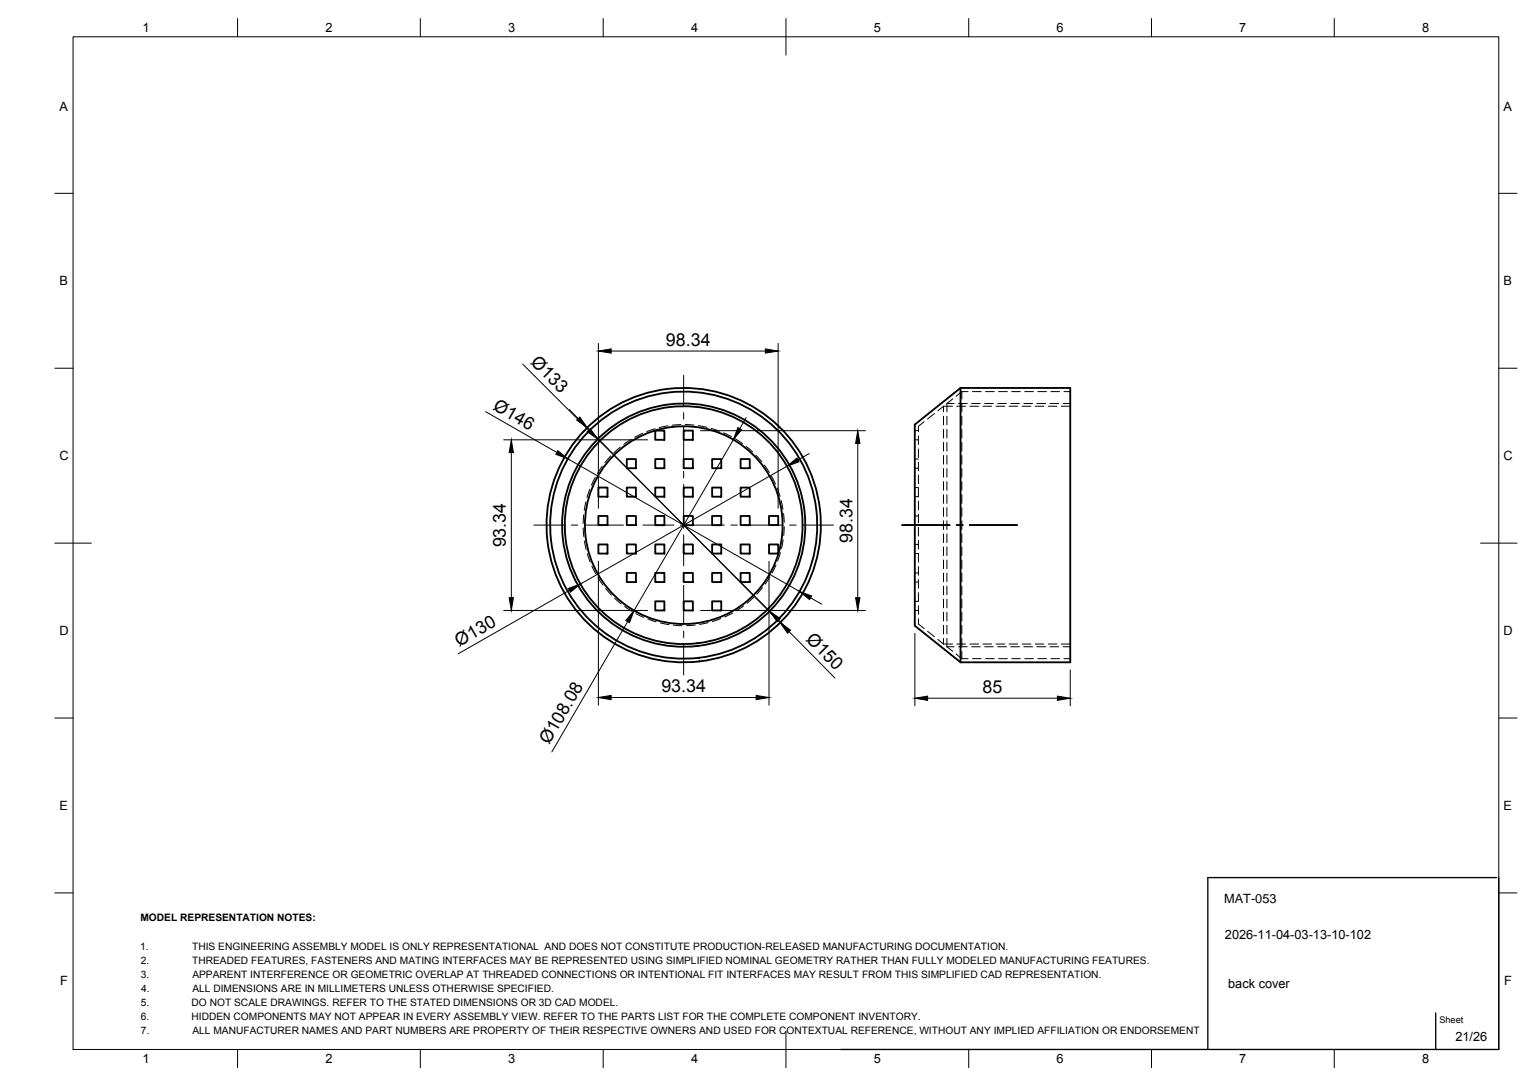
ISO-10303-21;
HEADER;
FILE_DESCRIPTION (('STEP AP214'),
    '1' );
FILE_NAME ('back cover.step',
    '2026-10-10T03:43:58',
    ( '' ),
    ( '' ),
    'SwSTEP 2.0',
    'SolidWorks 2026',
    '' );
FILE_SCHEMA (( 'AUTOMOTIVE_DESIGN' ));
ENDSEC;

DATA;
#6=DIRECTION ( 'NONE',  ( 0.000000000000000000, -1.000000000000000000, 0.000000000000000000 ) ) ;
#36=CARTESIAN_POINT ( 'NONE',  ( 0.000000000000000000, 0.000000000000000000, 0.000000000000000000 ) ) ;
#57=AXIS2_PLACEMENT_3D ( 'NONE', #19183, #8994, #35375 ) ;
#63=ORIENTED_EDGE ( 'NONE', *, *, #15028, .F. ) ;
#64=ORIENTED_EDGE ( 'NONE', *, *, #47335, .F. ) ;
#74=VECTOR ( 'NONE', #64267, 1000.000000000000000 ) ;
#81=CARTESIAN_POINT ( 'NONE',  ( -20.55634918610396866, 36.11269837220808654, 0.000000000000000000 ) ) ;
#91=CARTESIAN_POINT ( 'NONE',  ( 0.000000000000000000, 0.000000000000000000, 25.00000000000007816 ) ) ;
#96=DIRECTION ( 'NONE',  ( -0.000000000000000000, -0.000000000000000000, -1.000000000000000000 ) ) ;
#97=ORIENTED_EDGE ( 'NONE', *, *, #54272, .F. ) ;
#104=VECTOR ( 'NONE', #8568, 1000.000000000000000 ) ;
#111=VECTOR ( 'NONE', #38454, 1000.000000000000000 ) ;
#118=DIRECTION ( 'NONE',  ( -0.000000000000000000, -0.000000000000000000, -1.000000000000000000 ) ) ;
#120=ORIENTED_EDGE ( 'NONE', *, *, #64988, .T. ) ;
#150=EDGE_CURVE ( 'NONE', #43731, #18069, #10487, .T. ) ;
#166=AXIS2_PLACEMENT_3D ( 'NONE', #40198, #13463, #28960 ) ;
#171=VECTOR ( 'NONE', #36242, 1000.000000000000000 ) ;
#190=CARTESIAN_POINT ( 'NONE',  ( -31.11269837220812207, -26.11269837220801193, 0.000000000000000000 ) ) ;
#192=VERTEX_POINT ( 'NONE', #42509 ) ;
#195=FACE_BOUND ( 'NONE', #48020, .T. ) ;
#204=LINE ( 'NONE', #41148, #41347 ) ;
#234=EDGE_CURVE ( 'NONE', #1187, #8293, #15089, .T. ) ;
#287=LINE ( 'NONE', #43194, #50190 ) ;
#293=ORIENTED_EDGE ( 'NONE', *, *, #14607, .T. ) ;
#296=VECTOR ( 'NONE', #1863, 1000.000000000000000 ) ;
#300=FACE_OUTER_BOUND ( 'NONE', #57072, .T. ) ;
#306=AXIS2_PLACEMENT_3D ( 'NONE', #41965, #53186, #58819 ) ;
#322=ADVANCED_FACE ( 'NONE', ( #635 ), #43872, .F. ) ;
#327=VERTEX_POINT ( 'NONE', #60057 ) ;
#344=VECTOR ( 'NONE', #34891, 1000.000000000000000 ) ;
#349=DIRECTION ( 'NONE',  ( -1.000000000000000000, 0.000000000000000000, 0.000000000000000000 ) ) ;
#371=CARTESIAN_POINT ( 'NONE',  ( -20.55634918610396866, 31.11269837220809009, 0.000000000000000000 ) ) ;
#418=AXIS2_PLACEMENT_3D ( 'NONE', #49039, #43423, #65240 ) ;
#430=CARTESIAN_POINT ( 'NONE',  ( -20.55634918610403261, 0.000000000000000000, 2.000000000000000000 ) ) ;
#437=DIRECTION ( 'NONE',  ( 0.000000000000000000, 0.000000000000000000, 1.000000000000000000 ) ) ;
#440=DIRECTION ( 'NONE',  ( 0.000000000000000000, 1.000000000000000000, 0.000000000000000000 ) ) ;
#447=ORIENTED_EDGE ( 'NONE', *, *, #56885, .F. ) ;
#455=CARTESIAN_POINT ( 'NONE',  ( 15.55634918610400241, -15.55634918610406103, 85.00100000000000477 ) ) ;
#465=AXIS2_PLACEMENT_3D ( 'NONE', #65616, #23741, #6150 ) ;
#481=DIRECTION ( 'NONE',  ( 0.000000000000000000, 0.000000000000000000, 1.000000000000000000 ) ) ;
#522=VECTOR ( 'NONE', #50610, 1000.000000000000000 ) ;
#544=CARTESIAN_POINT ( 'NONE',  ( 6.375108774214766072E-14, 31.11269837220806167, 0.000000000000000000 ) ) ;
#553=CARTESIAN_POINT ( 'NONE',  ( -2.645453300864630819E-14, -15.55634918610403616, 2.000000000000001776 ) ) ;
#556=ADVANCED_FACE ( 'NONE', ( #43363 ), #46664, .F. ) ;
#557=DIRECTION ( 'NONE',  ( 0.000000000000000000, 1.000000000000000000, -0.000000000000000000 ) ) ;
#558=VECTOR ( 'NONE', #9205, 1000.000000000000000 ) ;
#565=LINE ( 'NONE', #27282, #37965 ) ;
#576=EDGE_LOOP ( 'NONE', ( #32786, #49878, #58567, #41798 ) ) ;
#578=CARTESIAN_POINT ( 'NONE',  ( -15.55634918610405748, -15.55634918610400774, 85.00100000000000477 ) ) ;
#588=EDGE_LOOP ( 'NONE', ( #66796, #38550, #24211, #31113 ) ) ;
#600=CARTESIAN_POINT ( 'NONE',  ( -7.329206686002009974E-14, -46.66904755831211560, 85.00100000000000477 ) ) ;
#607=ORIENTED_EDGE ( 'NONE', *, *, #30585, .F. ) ;
#613=EDGE_CURVE ( 'NONE', #67838, #27835, #64835, .T. ) ;
#632=EDGE_CURVE ( 'NONE', #26921, #4856, #48977, .T. ) ;
#635=FACE_OUTER_BOUND ( 'NONE', #24714, .T. ) ;
#643=ORIENTED_EDGE ( 'NONE', *, *, #36304, .T. ) ;
#661=DIRECTION ( 'NONE',  ( 0.000000000000000000, -1.000000000000000000, 0.000000000000000000 ) ) ;
#666=LINE ( 'NONE', #15804, #31702 ) ;
#730=FACE_OUTER_BOUND ( 'NONE', #7347, .T. ) ;
#790=EDGE_CURVE ( 'NONE', #8416, #11547, #57246, .T. ) ;
#801=ORIENTED_EDGE ( 'NONE', *, *, #53338, .F. ) ;
#827=DIRECTION ( 'NONE',  ( 0.000000000000000000, -1.000000000000000000, 0.000000000000000000 ) ) ;
#828=FACE_OUTER_BOUND ( 'NONE', #18462, .T. ) ;
#840=ORIENTED_EDGE ( 'NONE', *, *, #43108, .F. ) ;
#841=CARTESIAN_POINT ( 'NONE',  ( 0.000000000000000000, 0.000000000000000000, 85.00000000000000000 ) ) ;
#848=VECTOR ( 'NONE', #5552, 1000.000000000000000 ) ;
#877=ORIENTED_EDGE ( 'NONE', *, *, #51299, .F. ) ;
#882=DIRECTION ( 'NONE',  ( 0.000000000000000000, 1.000000000000000000, 0.000000000000000000 ) ) ;
#885=ORIENTED_EDGE ( 'NONE', *, *, #41118, .F. ) ;
#888=ORIENTED_EDGE ( 'NONE', *, *, #62836, .F. ) ;
#891=FACE_OUTER_BOUND ( 'NONE', #1268, .T. ) ;
#904=PLANE ( 'NONE',  #39037 ) ;
#906=DIRECTION ( 'NONE',  ( 1.000000000000000000, -0.000000000000000000, -0.000000000000000000 ) ) ;
#913=VERTEX_POINT ( 'NONE', #44161 ) ;
#920=CARTESIAN_POINT ( 'NONE',  ( 15.55634918610411610, 46.66904755831205875, 85.00100000000000477 ) ) ;
#931=DIRECTION ( 'NONE',  ( -1.000000000000000000, 0.000000000000000000, 0.000000000000000000 ) ) ;
#949=DIRECTION ( 'NONE',  ( 0.000000000000000000, 1.000000000000000000, -0.000000000000000000 ) ) ;
#958=VECTOR ( 'NONE', #53885, 1000.000000000000000 ) ;
#975=DIRECTION ( 'NONE',  ( 0.000000000000000000, 1.000000000000000000, -0.000000000000000000 ) ) ;
#984=CARTESIAN_POINT ( 'NONE',  ( -5.000000000000073719, -41.66904755831212270, 0.000000000000000000 ) ) ;
#993=ORIENTED_EDGE ( 'NONE', *, *, #35206, .T. ) ;
#1007=VECTOR ( 'NONE', #24608, 1000.000000000000000 ) ;
#1009=EDGE_CURVE ( 'NONE', #57581, #8542, #59993, .T. ) ;
#1021=EDGE_LOOP ( 'NONE', ( #20694, #3514, #16394, #42951 ) ) ;
#1035=VERTEX_POINT ( 'NONE', #14260 ) ;
#1047=CARTESIAN_POINT ( 'NONE',  ( 31.11269837220803325, -15.55634918610409656, 2.000000000000001776 ) ) ;
#1053=LINE ( 'NONE', #32712, #68406 ) ;
#1066=ORIENTED_EDGE ( 'NONE', *, *, #15157, .T. ) ;
#1079=CARTESIAN_POINT ( 'NONE',  ( -4.999999999999936939, 36.11269837220805812, 85.00100000000000477 ) ) ;
#1083=LINE ( 'NONE', #49599, #33421 ) ;
#1087=CARTESIAN_POINT ( 'NONE',  ( -51.66904755831212981, -15.55634918610397222, 0.000000000000000000 ) ) ;
#1089=ORIENTED_EDGE ( 'NONE', *, *, #65531, .F. ) ;
#1090=VECTOR ( 'NONE', #39346, 1000.000000000000000 ) ;
#1106=ORIENTED_EDGE ( 'NONE', *, *, #20088, .F. ) ;
#1122=LINE ( 'NONE', #17650, #64641 ) ;
#1141=LINE ( 'NONE', #39137, #57724 ) ;
#1164=EDGE_CURVE ( 'NONE', #53174, #39681, #69076, .T. ) ;
#1173=VECTOR ( 'NONE', #25176, 1000.000000000000000 ) ;
#1177=CARTESIAN_POINT ( 'NONE',  ( 10.55634918610400419, -10.55634918610406281, 2.000000000000001776 ) ) ;
#1178=LINE ( 'NONE', #22633, #24273 ) ;
#1187=VERTEX_POINT ( 'NONE', #69435 ) ;
#1190=SURFACE_STYLE_FILL_AREA ( #60284 ) ;
#1192=EDGE_CURVE ( 'NONE', #19369, #63634, #42702, .T. ) ;
#1203=DIRECTION ( 'NONE',  ( -1.000000000000000000, 0.000000000000000000, 0.000000000000000000 ) ) ;
#1226=CARTESIAN_POINT ( 'NONE',  ( -31.11269837220801193, 31.11269837220812207, 2.000000000000001776 ) ) ;
#1235=VERTEX_POINT ( 'NONE', #11731 ) ;
#1248=FACE_OUTER_BOUND ( 'NONE', #33448, .T. ) ;
#1249=ADVANCED_FACE ( 'NONE', ( #66278 ), #33203, .F. ) ;
#1250=FACE_BOUND ( 'NONE', #49319, .T. ) ;
#1268=EDGE_LOOP ( 'NONE', ( #11768, #41933, #16549, #1900 ) ) ;
#1271=VECTOR ( 'NONE', #7727, 1000.000000000000000 ) ;
#1283=EDGE_LOOP ( 'NONE', ( #47982, #4355, #44982, #36285 ) ) ;
#1293=DIRECTION ( 'NONE',  ( 1.000000000000000000, -0.000000000000000000, 0.000000000000000000 ) ) ;
#1326=PLANE ( 'NONE',  #5078 ) ;
#1335=VECTOR ( 'NONE', #46755, 1000.000000000000000 ) ;
#1344=DIRECTION ( 'NONE',  ( -0.000000000000000000, -0.000000000000000000, -1.000000000000000000 ) ) ;
#1346=DIRECTION ( 'NONE',  ( 1.000000000000000000, -0.000000000000000000, 0.000000000000000000 ) ) ;
#1349=EDGE_CURVE ( 'NONE', #50750, #8416, #55694, .T. ) ;
#1351=ORIENTED_EDGE ( 'NONE', *, *, #50161, .T. ) ;
#1361=DIRECTION ( 'NONE',  ( 0.000000000000000000, 0.000000000000000000, 1.000000000000000000 ) ) ;
#1381=EDGE_LOOP ( 'NONE', ( #20943, #1491, #51722, #43619 ) ) ;
#1386=AXIS2_PLACEMENT_3D ( 'NONE', #23783, #34697, #56132 ) ;
#1398=PLANE ( 'NONE',  #59758 ) ;
#1420=CARTESIAN_POINT ( 'NONE',  ( 10.55634918610400419, -15.55634918610406103, 85.00100000000000477 ) ) ;
#1446=DIRECTION ( 'NONE',  ( 1.000000000000000000, 0.000000000000000000, 0.000000000000000000 ) ) ;
#1451=CARTESIAN_POINT ( 'NONE',  ( -20.55634918610405748, -15.55634918610400774, 0.000000000000000000 ) ) ;
#1454=VERTEX_POINT ( 'NONE', #29656 ) ;
#1459=DIRECTION ( 'NONE',  ( 0.000000000000000000, -1.000000000000000000, 0.000000000000000000 ) ) ;
#1467=CARTESIAN_POINT ( 'NONE',  ( 41.66904755831212981, 15.55634918610394379, 0.000000000000000000 ) ) ;
#1482=ORIENTED_EDGE ( 'NONE', *, *, #22147, .F. ) ;
#1491=ORIENTED_EDGE ( 'NONE', *, *, #22147, .T. ) ;
#1534=ORIENTED_EDGE ( 'NONE', *, *, #38769, .T. ) ;
#1544=ORIENTED_EDGE ( 'NONE', *, *, #54272, .T. ) ;
#1582=DIRECTION ( 'NONE',  ( -0.000000000000000000, -1.000000000000000000, -0.000000000000000000 ) ) ;
#1608=CARTESIAN_POINT ( 'NONE',  ( 15.55634918610397399, -26.11269837220809364, 2.000000000000001776 ) ) ;
#1617=VERTEX_POINT ( 'NONE', #5168 ) ;
#1620=CARTESIAN_POINT ( 'NONE',  ( 10.55634918610411432, 51.66904755831205875, 85.00100000000000477 ) ) ;
#1635=LINE ( 'NONE', #12540, #16170 ) ;
#1653=ORIENTED_EDGE ( 'NONE', *, *, #26539, .T. ) ;
#1656=CARTESIAN_POINT ( 'NONE',  ( 31.11269837220800127, -31.11269837220812562, 2.000000000000001776 ) ) ;
#1657=DIRECTION ( 'NONE',  ( 0.000000000000000000, -0.000000000000000000, -1.000000000000000000 ) ) ;
#1672=AXIS2_PLACEMENT_3D ( 'NONE', #56432, #23047, #8255 ) ;
#1674=EDGE_CURVE ( 'NONE', #9968, #27957, #11131, .T. ) ;
#1729=DIRECTION ( 'NONE',  ( -0.000000000000000000, -0.000000000000000000, -1.000000000000000000 ) ) ;
#1731=ORIENTED_EDGE ( 'NONE', *, *, #59531, .F. ) ;
#1738=ORIENTED_EDGE ( 'NONE', *, *, #8963, .F. ) ;
#1759=ADVANCED_FACE ( 'NONE', ( #12190 ), #60716, .F. ) ;
#1764=DIRECTION ( 'NONE',  ( 0.000000000000000000, 0.000000000000000000, 1.000000000000000000 ) ) ;
#1768=EDGE_CURVE ( 'NONE', #27095, #38528, #55793, .T. ) ;
#1790=LINE ( 'NONE', #17961, #25329 ) ;
#1818=CARTESIAN_POINT ( 'NONE',  ( -5.767955557622883589E-14, -26.11269837220806522, 2.000000000000001776 ) ) ;
#1826=EDGE_CURVE ( 'NONE', #31701, #24549, #49803, .T. ) ;
#1853=DIRECTION ( 'NONE',  ( -1.000000000000000000, 0.000000000000000000, 0.000000000000000000 ) ) ;
#1863=DIRECTION ( 'NONE',  ( 0.000000000000000000, -1.000000000000000000, 0.000000000000000000 ) ) ;
#1888=VECTOR ( 'NONE', #8941, 1000.000000000000000 ) ;
#1894=CARTESIAN_POINT ( 'NONE',  ( 41.66904755831210849, -9.150666335777657423E-14, 85.00100000000000477 ) ) ;
#1900=ORIENTED_EDGE ( 'NONE', *, *, #46935, .F. ) ;
#1904=ORIENTED_EDGE ( 'NONE', *, *, #36060, .T. ) ;
#1909=EDGE_CURVE ( 'NONE', #62027, #63672, #20228, .T. ) ;
#1915=EDGE_CURVE ( 'NONE', #26889, #39680, #35031, .T. ) ;
#1916=ORIENTED_EDGE ( 'NONE', *, *, #8825, .T. ) ;
#1997=ORIENTED_EDGE ( 'NONE', *, *, #12232, .T. ) ;
#2018=VERTEX_POINT ( 'NONE', #25866 ) ;
#2020=CARTESIAN_POINT ( 'NONE',  ( 10.55634918610411432, 46.66904755831205875, 85.00100000000000477 ) ) ;
#2021=DIRECTION ( 'NONE',  ( -1.000000000000000000, 0.000000000000000000, 0.000000000000000000 ) ) ;
#2046=DIRECTION ( 'NONE',  ( -1.000000000000000000, 0.000000000000000000, 0.000000000000000000 ) ) ;
#2084=EDGE_CURVE ( 'NONE', #40853, #60572, #12105, .T. ) ;
#2088=ORIENTED_EDGE ( 'NONE', *, *, #49767, .F. ) ;
#2106=DIRECTION ( 'NONE',  ( 0.000000000000000000, -1.000000000000000000, 0.000000000000000000 ) ) ;
#2109=DIRECTION ( 'NONE',  ( 1.000000000000000000, -0.000000000000000000, 0.000000000000000000 ) ) ;
#2113=DIRECTION ( 'NONE',  ( -0.000000000000000000, -0.000000000000000000, -1.000000000000000000 ) ) ;
#2161=ORIENTED_EDGE ( 'NONE', *, *, #63382, .T. ) ;
#2162=LINE ( 'NONE', #13743, #57665 ) ;
#2168=LINE ( 'NONE', #45410, #29903 ) ;
#2172=EDGE_LOOP ( 'NONE', ( #17537, #12775, #56513, #41341 ) ) ;
#2175=LINE ( 'NONE', #18695, #68256 ) ;
#2187=DIRECTION ( 'NONE',  ( -1.000000000000000000, 0.000000000000000000, 0.000000000000000000 ) ) ;
#2188=DIRECTION ( 'NONE',  ( -1.000000000000000000, 0.000000000000000000, 0.000000000000000000 ) ) ;
#2213=LINE ( 'NONE', #32821, #63921 ) ;
#2216=ORIENTED_EDGE ( 'NONE', *, *, #20941, .T. ) ;
#2224=VECTOR ( 'NONE', #64142, 1000.000000000000000 ) ;
#2257=ORIENTED_EDGE ( 'NONE', *, *, #26764, .T. ) ;
#2258=PLANE ( 'NONE',  #31609 ) ;
#2265=CARTESIAN_POINT ( 'NONE',  ( -46.66904755831212981, -15.55634918610397222, 0.000000000000000000 ) ) ;
#2333=PLANE ( 'NONE',  #1386 ) ;
#2344=LINE ( 'NONE', #17101, #4229 ) ;
#2345=VECTOR ( 'NONE', #16431, 1000.000000000000000 ) ;
#2361=VECTOR ( 'NONE', #29823, 1000.000000000000000 ) ;
#2391=FACE_BOUND ( 'NONE', #20555, .T. ) ;
#2401=EDGE_CURVE ( 'NONE', #58133, #49065, #24667, .T. ) ;
#2426=CARTESIAN_POINT ( 'NONE',  ( 15.55634918610400241, -15.55634918610406103, 0.000000000000000000 ) ) ;
#2442=VECTOR ( 'NONE', #25225, 1000.000000000000000 ) ;
#2449=DIRECTION ( 'NONE',  ( 1.000000000000000000, -0.000000000000000000, 0.000000000000000000 ) ) ;
#2473=ORIENTED_EDGE ( 'NONE', *, *, #43442, .T. ) ;
#2482=EDGE_LOOP ( 'NONE', ( #8029, #97, #20347, #42967 ) ) ;
#2498=VECTOR ( 'NONE', #34813, 1000.000000000000000 ) ;
#2500=ORIENTED_EDGE ( 'NONE', *, *, #27204, .T. ) ;
#2502=ORIENTED_EDGE ( 'NONE', *, *, #48803, .F. ) ;
#2504=CIRCLE ( 'NONE', #11457, 66.50000000000000000 ) ;
#2517=CARTESIAN_POINT ( 'NONE',  ( -5.000000000000073719, -41.66904755831212270, 85.00100000000000477 ) ) ;
#2519=FACE_OUTER_BOUND ( 'NONE', #35690, .T. ) ;
#2538=ORIENTED_EDGE ( 'NONE', *, *, #32611, .T. ) ;
#2539=CARTESIAN_POINT ( 'NONE',  ( -5.767955557622883589E-14, -31.11269837220806878, 0.000000000000000000 ) ) ;
#2540=ADVANCED_FACE ( 'NONE', ( #63328 ), #42214, .F. ) ;
#2545=LINE ( 'NONE', #8521, #51988 ) ;
#2550=ORIENTED_EDGE ( 'NONE', *, *, #27368, .F. ) ;
#2570=ORIENTED_EDGE ( 'NONE', *, *, #11979, .T. ) ;
#2579=FACE_OUTER_BOUND ( 'NONE', #67824, .T. ) ;
#2590=CARTESIAN_POINT ( 'NONE',  ( 41.66904755831210849, 4.999999999999909406, 2.000000000000001776 ) ) ;
#2629=PLANE ( 'NONE',  #1672 ) ;
#2631=DIRECTION ( 'NONE',  ( -1.000000000000000000, 0.000000000000000000, 0.000000000000000000 ) ) ;
#2645=PLANE ( 'NONE',  #51441 ) ;
#2651=VERTEX_POINT ( 'NONE', #22484 ) ;
#2660=DIRECTION ( 'NONE',  ( -0.000000000000000000, -0.000000000000000000, -1.000000000000000000 ) ) ;
#2670=LINE ( 'NONE', #30103, #1173 ) ;
#2689=ORIENTED_EDGE ( 'NONE', *, *, #47335, .T. ) ;
#2701=VECTOR ( 'NONE', #8433, 1000.000000000000000 ) ;
#2704=VECTOR ( 'NONE', #14100, 999.9999999999998863 ) ;
#2716=ORIENTED_EDGE ( 'NONE', *, *, #45081, .F. ) ;
#2723=LINE ( 'NONE', #35425, #51095 ) ;
#2726=ORIENTED_EDGE ( 'NONE', *, *, #15157, .F. ) ;
#2732=ORIENTED_EDGE ( 'NONE', *, *, #31234, .T. ) ;
#2735=FACE_BOUND ( 'NONE', #45270, .T. ) ;
#2736=VECTOR ( 'NONE', #37672, 1000.000000000000000 ) ;
#2764=FACE_OUTER_BOUND ( 'NONE', #14655, .T. ) ;
#2783=VECTOR ( 'NONE', #29904, 1000.000000000000000 ) ;
#2789=CARTESIAN_POINT ( 'NONE',  ( -31.11269837220801193, 31.11269837220812207, 2.000000000000001776 ) ) ;
#2803=CARTESIAN_POINT ( 'NONE',  ( 15.55634918610411610, 46.66904755831205875, 0.000000000000000000 ) ) ;
#2836=DIRECTION ( 'NONE',  ( -1.000000000000000000, 0.000000000000000000, 0.000000000000000000 ) ) ;
#2837=EDGE_CURVE ( 'NONE', #34252, #12488, #63161, .T. ) ;
#2847=AXIS2_PLACEMENT_3D ( 'NONE', #55235, #19692, #19004 ) ;
#2860=ADVANCED_FACE ( 'NONE', ( #52591 ), #57538, .F. ) ;
#2864=CARTESIAN_POINT ( 'NONE',  ( -20.55634918610403261, 5.000000000000028422, 85.00100000000000477 ) ) ;
#2865=ADVANCED_FACE ( 'NONE', ( #24240 ), #28817, .F. ) ;
#2871=CARTESIAN_POINT ( 'NONE',  ( 31.11269837220806522, -6.375108774214766072E-14, 0.000000000000000000 ) ) ;
#2886=AXIS2_PLACEMENT_3D ( 'NONE', #12370, #66210, #45064 ) ;
#2899=DIRECTION ( 'NONE',  ( -0.000000000000000000, -0.000000000000000000, -1.000000000000000000 ) ) ;
#2908=PLANE ( 'NONE',  #63965 ) ;
#2921=CARTESIAN_POINT ( 'NONE',  ( -5.767955557622883589E-14, -26.11269837220806522, 0.000000000000000000 ) ) ;
#2924=DIRECTION ( 'NONE',  ( 1.000000000000000000, 0.000000000000000000, 0.000000000000000000 ) ) ;
#2926=EDGE_CURVE ( 'NONE', #61056, #43813, #64883, .T. ) ;
#2998=CARTESIAN_POINT ( 'NONE',  ( 46.66904755831207297, -15.55634918610412853, 85.00100000000000477 ) ) ;
#3003=DIRECTION ( 'NONE',  ( 0.000000000000000000, -1.000000000000000000, 0.000000000000000000 ) ) ;
#3006=ORIENTED_EDGE ( 'NONE', *, *, #12801, .T. ) ;
#3014=EDGE_CURVE ( 'NONE', #26941, #30210, #39202, .T. ) ;
#3043=DIRECTION ( 'NONE',  ( -0.000000000000000000, -0.000000000000000000, -1.000000000000000000 ) ) ;
#3073=LINE ( 'NONE', #24536, #42722 ) ;
#3074=LINE ( 'NONE', #56888, #2442 ) ;
#3090=ORIENTED_EDGE ( 'NONE', *, *, #38328, .F. ) ;
#3093=ADVANCED_FACE ( 'NONE', ( #8228 ), #9260, .F. ) ;
#3094=AXIS2_PLACEMENT_3D ( 'NONE', #16311, #33194, #481 ) ;
#3103=DIRECTION ( 'NONE',  ( 0.000000000000000000, 1.000000000000000000, 0.000000000000000000 ) ) ;
#3141=AXIS2_PLACEMENT_3D ( 'NONE', #68861, #20685, #1657 ) ;
#3154=DIRECTION ( 'NONE',  ( -0.000000000000000000, -0.000000000000000000, -1.000000000000000000 ) ) ;
#3173=EDGE_CURVE ( 'NONE', #53918, #30808, #10975, .T. ) ;
#3178=ADVANCED_FACE ( 'NONE', ( #37029 ), #47913, .F. ) ;
#3196=DIRECTION ( 'NONE',  ( 0.000000000000000000, 0.000000000000000000, 1.000000000000000000 ) ) ;
#3198=ORIENTED_EDGE ( 'NONE', *, *, #22337, .F. ) ;
#3216=CARTESIAN_POINT ( 'NONE',  ( -15.55634918610400597, 15.55634918610405748, 85.00100000000000477 ) ) ;
#3219=DIRECTION ( 'NONE',  ( -1.000000000000000000, 0.000000000000000000, 0.000000000000000000 ) ) ;
#3244=ORIENTED_EDGE ( 'NONE', *, *, #60272, .T. ) ;
#3255=CARTESIAN_POINT ( 'NONE',  ( -31.11269837220812207, -31.11269837220801193, 85.00100000000000477 ) ) ;
#3258=DIRECTION ( 'NONE',  ( 0.000000000000000000, 0.000000000000000000, 1.000000000000000000 ) ) ;
#3267=PLANE ( 'NONE',  #34590 ) ;
#3307=DIRECTION ( 'NONE',  ( -1.000000000000000000, 0.000000000000000000, 0.000000000000000000 ) ) ;
#3312=DIRECTION ( 'NONE',  ( 0.000000000000000000, 0.000000000000000000, -1.000000000000000000 ) ) ;
#3322=DIRECTION ( 'NONE',  ( 0.000000000000000000, 1.000000000000000000, -0.000000000000000000 ) ) ;
#3344=EDGE_CURVE ( 'NONE', #327, #48751, #18345, .T. ) ;
#3346=VERTEX_POINT ( 'NONE', #65497 ) ;
#3356=ORIENTED_EDGE ( 'NONE', *, *, #64407, .F. ) ;
#3367=CARTESIAN_POINT ( 'NONE',  ( -2.645453300864630819E-14, -15.55634918610403616, 0.000000000000000000 ) ) ;
#3399=EDGE_CURVE ( 'NONE', #16538, #26941, #22579, .T. ) ;
#3426=FACE_BOUND ( 'NONE', #67273, .T. ) ;
#3442=DIRECTION ( 'NONE',  ( 1.000000000000000000, -0.000000000000000000, 0.000000000000000000 ) ) ;
#3453=ORIENTED_EDGE ( 'NONE', *, *, #28604, .F. ) ;
#3465=DIRECTION ( 'NONE',  ( -0.000000000000000000, -1.000000000000000000, -0.000000000000000000 ) ) ;
#3482=EDGE_CURVE ( 'NONE', #32392, #65236, #45072, .T. ) ;
#3491=VECTOR ( 'NONE', #39909, 1000.000000000000000 ) ;
#3514=ORIENTED_EDGE ( 'NONE', *, *, #60185, .T. ) ;
#3518=FACE_OUTER_BOUND ( 'NONE', #5864, .T. ) ;
#3535=PLANE ( 'NONE',  #7568 ) ;
#3541=ORIENTED_EDGE ( 'NONE', *, *, #3648, .T. ) ;
#3544=DIRECTION ( 'NONE',  ( 1.000000000000000000, -0.000000000000000000, -0.000000000000000000 ) ) ;
#3603=FACE_OUTER_BOUND ( 'NONE', #44316, .T. ) ;
#3621=LINE ( 'NONE', #51125, #64131 ) ;
#3625=VERTEX_POINT ( 'NONE', #50237 ) ;
#3626=FACE_OUTER_BOUND ( 'NONE', #64552, .T. ) ;
#3636=AXIS2_PLACEMENT_3D ( 'NONE', #21413, #38283, #65379 ) ;
#3646=ORIENTED_EDGE ( 'NONE', *, *, #5690, .T. ) ;
#3648=EDGE_CURVE ( 'NONE', #15461, #1035, #69111, .T. ) ;
#3677=DIRECTION ( 'NONE',  ( 0.000000000000000000, 0.000000000000000000, 1.000000000000000000 ) ) ;
#3729=SHAPE_DEFINITION_REPRESENTATION ( #23215, #36585 ) ;
#3742=AXIS2_PLACEMENT_3D ( 'NONE', #59163, #32448, #64805 ) ;
#3747=ADVANCED_FACE ( 'NONE', ( #45514 ), #66998, .F. ) ;
#3767=FACE_OUTER_BOUND ( 'NONE', #30666, .T. ) ;
#3805=AXIS2_PLACEMENT_3D ( 'NONE', #7710, #9695, #9340 ) ;
#3817=EDGE_CURVE ( 'NONE', #2651, #47695, #50454, .T. ) ;
#3856=CARTESIAN_POINT ( 'NONE',  ( -31.11269837220809364, -15.55634918610397754, 2.000000000000001776 ) ) ;
#3879=ORIENTED_EDGE ( 'NONE', *, *, #36691, .F. ) ;
#3914=VERTEX_POINT ( 'NONE', #8237 ) ;
#3951=CARTESIAN_POINT ( 'NONE',  ( -20.55634918610411077, -46.66904755831208718, 0.000000000000000000 ) ) ;
#3968=VERTEX_POINT ( 'NONE', #47233 ) ;
#3970=LINE ( 'NONE', #25087, #24901 ) ;
#3981=EDGE_CURVE ( 'NONE', #51672, #48751, #63078, .T. ) ;
#4012=ORIENTED_EDGE ( 'NONE', *, *, #21210, .F. ) ;
#4037=ORIENTED_EDGE ( 'NONE', *, *, #63361, .T. ) ;
#4041=LINE ( 'NONE', #62439, #56806 ) ;
#4048=CARTESIAN_POINT ( 'NONE',  ( 15.55634918610396511, -46.66904755831214402, 85.00100000000000477 ) ) ;
#4063=ORIENTED_EDGE ( 'NONE', *, *, #23203, .F. ) ;
#4085=ORIENTED_EDGE ( 'NONE', *, *, #15028, .T. ) ;
#4086=VECTOR ( 'NONE', #31580, 1000.000000000000000 ) ;
#4096=VECTOR ( 'NONE', #43353, 1000.000000000000000 ) ;
#4100=DIRECTION ( 'NONE',  ( 0.000000000000000000, 1.000000000000000000, 0.000000000000000000 ) ) ;
#4105=DIRECTION ( 'NONE',  ( -1.000000000000000000, 0.000000000000000000, 0.000000000000000000 ) ) ;
#4106=DIRECTION ( 'NONE',  ( 1.000000000000000000, -0.000000000000000000, -0.000000000000000000 ) ) ;
#4115=CARTESIAN_POINT ( 'NONE',  ( -2.645453300864630819E-14, -10.55634918610403439, 0.000000000000000000 ) ) ;
#4123=EDGE_CURVE ( 'NONE', #25726, #42920, #11325, .T. ) ;
#4130=ORIENTED_EDGE ( 'NONE', *, *, #28912, .F. ) ;
#4151=CARTESIAN_POINT ( 'NONE',  ( 10.55634918610400419, -15.55634918610406103, 0.000000000000000000 ) ) ;
#4161=ORIENTED_EDGE ( 'NONE', *, *, #14337, .F. ) ;
#4177=VECTOR ( 'NONE', #31591, 1000.000000000000000 ) ;
#4190=EDGE_LOOP ( 'NONE', ( #41859, #2257, #52891, #50930 ) ) ;
#4192=AXIS2_PLACEMENT_3D ( 'NONE', #59060, #5260, #59405 ) ;
#4201=ORIENTED_EDGE ( 'NONE', *, *, #38594, .T. ) ;
#4208=EDGE_CURVE ( 'NONE', #27210, #48270, #46816, .T. ) ;
#4229=VECTOR ( 'NONE', #1293, 1000.000000000000000 ) ;
#4237=DIRECTION ( 'NONE',  ( 0.000000000000000000, -0.000000000000000000, -1.000000000000000000 ) ) ;
#4279=ADVANCED_FACE ( 'NONE', ( #36613 ), #64030, .F. ) ;
#4295=CARTESIAN_POINT ( 'NONE',  ( 74.99999999999998579, 9.184850993605147156E-15, 85.00000000000000000 ) ) ;
#4314=EDGE_LOOP ( 'NONE', ( #18950, #35368, #65861, #24670 ) ) ;
#4316=ORIENTED_EDGE ( 'NONE', *, *, #40336, .F. ) ;
#4326=LINE ( 'NONE', #10273, #68947 ) ;
#4327=EDGE_CURVE ( 'NONE', #69014, #18870, #37986, .T. ) ;
#4355=ORIENTED_EDGE ( 'NONE', *, *, #12645, .F. ) ;
#4358=ORIENTED_EDGE ( 'NONE', *, *, #49839, .F. ) ;
#4378=VECTOR ( 'NONE', #2631, 1000.000000000000000 ) ;
#4405=ORIENTED_EDGE ( 'NONE', *, *, #49887, .F. ) ;
#4424=CARTESIAN_POINT ( 'NONE',  ( -31.11269837220812207, -31.11269837220801193, 0.000000000000000000 ) ) ;
#4433=ORIENTED_EDGE ( 'NONE', *, *, #30921, .F. ) ;
#4447=PLANE ( 'NONE',  #28287 ) ;
#4457=CARTESIAN_POINT ( 'NONE',  ( 26.11269837220806167, 0.000000000000000000, 2.000000000000000000 ) ) ;
#4464=PLANE ( 'NONE',  #60927 ) ;
#4471=ORIENTED_EDGE ( 'NONE', *, *, #14219, .T. ) ;
#4472=ORIENTED_EDGE ( 'NONE', *, *, #53094, .F. ) ;
#4476=PLANE ( 'NONE',  #54164 ) ;
#4486=VERTEX_POINT ( 'NONE', #16788 ) ;
#4494=CARTESIAN_POINT ( 'NONE',  ( 0.000000000000000000, 0.000000000000000000, 25.00000000000007816 ) ) ;
#4524=CARTESIAN_POINT ( 'NONE',  ( 41.66904755831210849, -9.150666335777657423E-14, 85.00100000000000477 ) ) ;
#4532=ORIENTED_EDGE ( 'NONE', *, *, #64291, .T. ) ;
#4542=DIRECTION ( 'NONE',  ( -1.000000000000000000, 0.000000000000000000, 0.000000000000000000 ) ) ;
#4547=DIRECTION ( 'NONE',  ( -0.000000000000000000, -1.000000000000000000, -0.000000000000000000 ) ) ;
#4550=ORIENTED_EDGE ( 'NONE', *, *, #22704, .T. ) ;
#4555=LINE ( 'NONE', #14764, #53364 ) ;
#4563=VERTEX_POINT ( 'NONE', #16454 ) ;
#4570=DIRECTION ( 'NONE',  ( 0.000000000000000000, -1.000000000000000000, 0.000000000000000000 ) ) ;
#4580=CARTESIAN_POINT ( 'NONE',  ( -15.55634918610411077, -41.66904755831209428, 85.00100000000000477 ) ) ;
#4596=VERTEX_POINT ( 'NONE', #55118 ) ;
#4611=EDGE_CURVE ( 'NONE', #58000, #22638, #49131, .T. ) ;
#4613=ORIENTED_EDGE ( 'NONE', *, *, #50509, .T. ) ;
#4677=DIRECTION ( 'NONE',  ( 0.000000000000000000, 0.000000000000000000, 1.000000000000000000 ) ) ;
#4679=DIRECTION ( 'NONE',  ( -0.000000000000000000, -0.000000000000000000, -1.000000000000000000 ) ) ;
#4701=EDGE_CURVE ( 'NONE', #37117, #10376, #11608, .T. ) ;
#4710=DIRECTION ( 'NONE',  ( -0.000000000000000000, -0.000000000000000000, -1.000000000000000000 ) ) ;
#4740=EDGE_CURVE ( 'NONE', #60572, #16162, #27167, .T. ) ;
#4743=DIRECTION ( 'NONE',  ( 0.000000000000000000, -1.000000000000000000, 0.000000000000000000 ) ) ;
#4751=( NAMED_UNIT ( * ) PLANE_ANGLE_UNIT ( ) SI_UNIT ( $, .RADIAN. ) );
#4765=CARTESIAN_POINT ( 'NONE',  ( 31.11269837220809364, 20.55634918610396866, 0.000000000000000000 ) ) ;
#4778=CARTESIAN_POINT ( 'NONE',  ( 31.11269837220803325, -15.55634918610409656, 2.000000000000001776 ) ) ;
#4819=CARTESIAN_POINT ( 'NONE',  ( -36.11269837220801548, 36.11269837220812207, 0.000000000000000000 ) ) ;
#4823=AXIS2_PLACEMENT_3D ( 'NONE', #600, #43844, #5866 ) ;
#4855=DIRECTION ( 'NONE',  ( 0.000000000000000000, 0.000000000000000000, 1.000000000000000000 ) ) ;
#4856=VERTEX_POINT ( 'NONE', #37997 ) ;
#4872=FACE_OUTER_BOUND ( 'NONE', #46601, .T. ) ;
#4927=DIRECTION ( 'NONE',  ( -0.000000000000000000, -0.000000000000000000, -1.000000000000000000 ) ) ;
#4929=ORIENTED_EDGE ( 'NONE', *, *, #43895, .F. ) ;
#4933=ORIENTED_EDGE ( 'NONE', *, *, #26432, .T. ) ;
#4954=CARTESIAN_POINT ( 'NONE',  ( -20.55634918610408945, -31.11269837220804035, 0.000000000000000000 ) ) ;
#4958=ORIENTED_EDGE ( 'NONE', *, *, #24011, .F. ) ;
#4968=LINE ( 'NONE', #27107, #33681 ) ;
#4978=CARTESIAN_POINT ( 'NONE',  ( -5.000000000000058620, -31.11269837220806878, 2.000000000000000000 ) ) ;
#4995=PLANE ( 'NONE',  #37706 ) ;
#5030=VERTEX_POINT ( 'NONE', #43954 ) ;
#5041=ORIENTED_EDGE ( 'NONE', *, *, #67906, .F. ) ;
#5060=CARTESIAN_POINT ( 'NONE',  ( 72.99999999999998579, 8.939921633775675282E-15, 85.00000000000000000 ) ) ;
#5078=AXIS2_PLACEMENT_3D ( 'NONE', #60418, #29110, #49145 ) ;
#5092=EDGE_CURVE ( 'NONE', #3346, #26889, #39741, .T. ) ;
#5104=DIRECTION ( 'NONE',  ( -0.000000000000000000, -0.000000000000000000, -1.000000000000000000 ) ) ;
#5106=ORIENTED_EDGE ( 'NONE', *, *, #51386, .T. ) ;
#5117=ORIENTED_EDGE ( 'NONE', *, *, #39806, .F. ) ;
#5124=LINE ( 'NONE', #4778, #49873 ) ;
#5126=VECTOR ( 'NONE', #63857, 1000.000000000000000 ) ;
#5139=FACE_BOUND ( 'NONE', #5452, .T. ) ;
#5159=CYLINDRICAL_SURFACE ( 'NONE', #24851, 65.00000000000000000 ) ;
#5164=DIRECTION ( 'NONE',  ( -0.000000000000000000, -1.000000000000000000, -0.000000000000000000 ) ) ;
#5168=CARTESIAN_POINT ( 'NONE',  ( -15.55634918610400597, 20.55634918610405748, 2.000000000000001776 ) ) ;
#5179=VECTOR ( 'NONE', #22746, 1000.000000000000000 ) ;
#5188=DIRECTION ( 'NONE',  ( -1.000000000000000000, 0.000000000000000000, 0.000000000000000000 ) ) ;
#5194=CARTESIAN_POINT ( 'NONE',  ( -15.55634918610400597, 20.55634918610405748, 85.00100000000000477 ) ) ;
#5196=DIRECTION ( 'NONE',  ( 0.000000000000000000, 1.000000000000000000, 0.000000000000000000 ) ) ;
#5215=LINE ( 'NONE', #21057, #64490 ) ;
#5217=CARTESIAN_POINT ( 'NONE',  ( 46.66904755831210139, 4.999999999999909406, 85.00100000000000477 ) ) ;
#5222=DIRECTION ( 'NONE',  ( 0.000000000000000000, -0.000000000000000000, -1.000000000000000000 ) ) ;
#5243=EDGE_LOOP ( 'NONE', ( #2473, #20569, #48322, #43568 ) ) ;
#5245=EDGE_CURVE ( 'NONE', #45779, #42920, #25311, .T. ) ;
#5255=ORIENTED_EDGE ( 'NONE', *, *, #32277, .F. ) ;
#5260=DIRECTION ( 'NONE',  ( 1.000000000000000000, 0.000000000000000000, 0.000000000000000000 ) ) ;
#5264=EDGE_LOOP ( 'NONE', ( #19487, #7410, #68230, #42287 ) ) ;
#5267=ORIENTED_EDGE ( 'NONE', *, *, #18972, .F. ) ;
#5280=VECTOR ( 'NONE', #47775, 1000.000000000000000 ) ;
#5285=CARTESIAN_POINT ( 'NONE',  ( 41.66904755831212981, 15.55634918610394379, 2.000000000000001776 ) ) ;
#5300=EDGE_CURVE ( 'NONE', #24137, #58000, #24268, .T. ) ;
#5303=EDGE_LOOP ( 'NONE', ( #9494, #46522, #52950, #1731 ) ) ;
#5307=EDGE_CURVE ( 'NONE', #1035, #54490, #5215, .T. ) ;
#5346=VERTEX_POINT ( 'NONE', #26674 ) ;
#5373=VECTOR ( 'NONE', #9109, 1000.000000000000000 ) ;
#5385=CARTESIAN_POINT ( 'NONE',  ( -5.000000000000026645, -10.55634918610403439, 85.00100000000000477 ) ) ;
#5391=LINE ( 'NONE', #69408, #29896 ) ;
#5395=DIRECTION ( 'NONE',  ( 0.000000000000000000, 0.000000000000000000, -1.000000000000000000 ) ) ;
#5403=DIRECTION ( 'NONE',  ( 1.000000000000000000, 0.000000000000000000, 0.000000000000000000 ) ) ;
#5417=CARTESIAN_POINT ( 'NONE',  ( 6.375108774214766072E-14, 31.11269837220806167, 2.000000000000001776 ) ) ;
#5425=VECTOR ( 'NONE', #3154, 1000.000000000000000 ) ;
#5444=EDGE_CURVE ( 'NONE', #24127, #27835, #16111, .T. ) ;
#5452=EDGE_LOOP ( 'NONE', ( #67645, #57659, #47326, #4085 ) ) ;
#5482=FACE_BOUND ( 'NONE', #19895, .T. ) ;
#5483=EDGE_CURVE ( 'NONE', #40273, #57346, #32640, .T. ) ;
#5491=EDGE_LOOP ( 'NONE', ( #5106, #24890, #59631, #12168 ) ) ;
#5516=CARTESIAN_POINT ( 'NONE',  ( 6.375108774214766072E-14, 31.11269837220806167, 85.00100000000000477 ) ) ;
#5530=DIRECTION ( 'NONE',  ( 0.000000000000000000, -0.000000000000000000, -1.000000000000000000 ) ) ;
#5547=ADVANCED_FACE ( 'NONE', ( #6604 ), #28049, .F. ) ;
#5552=DIRECTION ( 'NONE',  ( -0.000000000000000000, -0.000000000000000000, -1.000000000000000000 ) ) ;
#5567=EDGE_CURVE ( 'NONE', #17255, #41880, #27700, .T. ) ;
#5594=LINE ( 'NONE', #27394, #28903 ) ;
#5600=LINE ( 'NONE', #27054, #48745 ) ;
#5602=VERTEX_POINT ( 'NONE', #34738 ) ;
#5603=ORIENTED_EDGE ( 'NONE', *, *, #8812, .T. ) ;
#5610=ORIENTED_EDGE ( 'NONE', *, *, #11689, .T. ) ;
#5662=LINE ( 'NONE', #55603, #65111 ) ;
#5667=ORIENTED_EDGE ( 'NONE', *, *, #47398, .F. ) ;
#5669=ORIENTED_EDGE ( 'NONE', *, *, #18594, .F. ) ;
#5690=EDGE_CURVE ( 'NONE', #17818, #30657, #5124, .T. ) ;
#5704=FACE_OUTER_BOUND ( 'NONE', #22344, .T. ) ;
#5715=ORIENTED_EDGE ( 'NONE', *, *, #45581, .T. ) ;
#5719=VERTEX_POINT ( 'NONE', #63531 ) ;
#5725=VECTOR ( 'NONE', #2109, 1000.000000000000000 ) ;
#5729=CARTESIAN_POINT ( 'NONE',  ( 46.66904755831210139, -9.150666335777657423E-14, 2.000000000000001776 ) ) ;
#5738=FACE_OUTER_BOUND ( 'NONE', #46135, .T. ) ;
#5743=VECTOR ( 'NONE', #25173, 1000.000000000000000 ) ;
#5748=DIRECTION ( 'NONE',  ( 0.000000000000000000, -0.000000000000000000, -1.000000000000000000 ) ) ;
#5761=EDGE_CURVE ( 'NONE', #56407, #18138, #10395, .T. ) ;
#5765=VERTEX_POINT ( 'NONE', #20272 ) ;
#5783=CARTESIAN_POINT ( 'NONE',  ( -4.999999999999936939, 36.11269837220805812, 0.000000000000000000 ) ) ;
#5791=DIRECTION ( 'NONE',  ( 1.000000000000000000, -0.000000000000000000, 0.000000000000000000 ) ) ;
#5798=ORIENTED_EDGE ( 'NONE', *, *, #18197, .T. ) ;
#5817=DIRECTION ( 'NONE',  ( 0.000000000000000000, 0.000000000000000000, 1.000000000000000000 ) ) ;
#5836=ORIENTED_EDGE ( 'NONE', *, *, #11076, .F. ) ;
#5842=LINE ( 'NONE', #43818, #8720 ) ;
#5848=DIRECTION ( 'NONE',  ( 1.000000000000000000, -0.000000000000000000, 0.000000000000000000 ) ) ;
#5851=EDGE_CURVE ( 'NONE', #62932, #32718, #68792, .T. ) ;
#5852=ORIENTED_EDGE ( 'NONE', *, *, #18118, .T. ) ;
#5863=DIRECTION ( 'NONE',  ( 0.000000000000000000, 0.000000000000000000, 1.000000000000000000 ) ) ;
#5864=EDGE_LOOP ( 'NONE', ( #18136, #41745, #25263, #35049 ) ) ;
#5866=DIRECTION ( 'NONE',  ( 0.000000000000000000, -0.000000000000000000, -1.000000000000000000 ) ) ;
#5876=EDGE_CURVE ( 'NONE', #13372, #34620, #52620, .T. ) ;
#5878=CARTESIAN_POINT ( 'NONE',  ( 15.55634918610396511, -46.66904755831214402, 2.000000000000001776 ) ) ;
#5888=DIRECTION ( 'NONE',  ( -0.000000000000000000, -1.000000000000000000, -0.000000000000000000 ) ) ;
#5902=CARTESIAN_POINT ( 'NONE',  ( -5.767955557622883589E-14, -31.11269837220806878, 85.00100000000000477 ) ) ;
#5912=ORIENTED_EDGE ( 'NONE', *, *, #51572, .F. ) ;
#5942=DIRECTION ( 'NONE',  ( -0.000000000000000000, -0.000000000000000000, -1.000000000000000000 ) ) ;
#5945=ORIENTED_EDGE ( 'NONE', *, *, #16520, .T. ) ;
#5967=EDGE_LOOP ( 'NONE', ( #34676, #50085, #29193, #40551 ) ) ;
#5977=CARTESIAN_POINT ( 'NONE',  ( -66.50000000000000000, 8.143901214329899974E-15, 85.00000000000000000 ) ) ;
#5978=ORIENTED_EDGE ( 'NONE', *, *, #5245, .F. ) ;
#5981=ORIENTED_EDGE ( 'NONE', *, *, #61492, .F. ) ;
#5983=VECTOR ( 'NONE', #67059, 1000.000000000000000 ) ;
#5990=DIRECTION ( 'NONE',  ( 0.6246950475544236214, 0.000000000000000000, 0.7808688094430308313 ) ) ;
#6007=FACE_OUTER_BOUND ( 'NONE', #40693, .T. ) ;
#6023=DIRECTION ( 'NONE',  ( 0.000000000000000000, 0.000000000000000000, 1.000000000000000000 ) ) ;
#6032=CIRCLE ( 'NONE', #418, 72.99999999999998579 ) ;
#6073=DIRECTION ( 'NONE',  ( -1.000000000000000000, 0.000000000000000000, 0.000000000000000000 ) ) ;
#6103=EDGE_CURVE ( 'NONE', #19020, #46372, #57484, .T. ) ;
#6114=EDGE_LOOP ( 'NONE', ( #32174, #38694, #18164, #14461 ) ) ;
#6130=VECTOR ( 'NONE', #23542, 1000.000000000000000 ) ;
#6142=CARTESIAN_POINT ( 'NONE',  ( 10.55634918610406281, 15.55634918610400241, 0.000000000000000000 ) ) ;
#6150=DIRECTION ( 'NONE',  ( 0.000000000000000000, 0.000000000000000000, 1.000000000000000000 ) ) ;
#6167=FACE_BOUND ( 'NONE', #54986, .T. ) ;
#6176=VECTOR ( 'NONE', #2021, 1000.000000000000000 ) ;
#6212=LINE ( 'NONE', #66033, #10927 ) ;
#6241=CONICAL_SURFACE ( 'NONE', #62393, 73.43826238111391547, 0.6747409422235518539 ) ;
#6253=ORIENTED_EDGE ( 'NONE', *, *, #37228, .F. ) ;
#6254=LINE ( 'NONE', #65360, #24437 ) ;
#6257=ORIENTED_EDGE ( 'NONE', *, *, #45589, .F. ) ;
#6282=CARTESIAN_POINT ( 'NONE',  ( -20.55634918610400419, 20.55634918610405748, 0.000000000000000000 ) ) ;
#6283=DIRECTION ( 'NONE',  ( -0.000000000000000000, -0.000000000000000000, -1.000000000000000000 ) ) ;
#6296=LINE ( 'NONE', #21431, #27776 ) ;
#6298=CARTESIAN_POINT ( 'NONE',  ( -15.55634918610408945, -26.11269837220804035, 2.000000000000001776 ) ) ;
#6301=LINE ( 'NONE', #17555, #9469 ) ;
#6312=ORIENTED_EDGE ( 'NONE', *, *, #52411, .F. ) ;
#6324=VECTOR ( 'NONE', #43029, 1000.000000000000000 ) ;
#6326=DIRECTION ( 'NONE',  ( -0.000000000000000000, -0.000000000000000000, -1.000000000000000000 ) ) ;
#6370=DIRECTION ( 'NONE',  ( -1.000000000000000000, 0.000000000000000000, 0.000000000000000000 ) ) ;
#6398=DIRECTION ( 'NONE',  ( 1.000000000000000000, -0.000000000000000000, -0.000000000000000000 ) ) ;
#6414=ORIENTED_EDGE ( 'NONE', *, *, #3817, .T. ) ;
#6432=DIRECTION ( 'NONE',  ( -0.000000000000000000, -0.000000000000000000, -1.000000000000000000 ) ) ;
#6502=EDGE_LOOP ( 'NONE', ( #46809, #4929, #29957, #22277 ) ) ;
#6511=EDGE_CURVE ( 'NONE', #37709, #13713, #64309, .T. ) ;
#6520=ADVANCED_FACE ( 'NONE', ( #4872 ), #68881, .F. ) ;
#6529=CARTESIAN_POINT ( 'NONE',  ( -7.329206686002009974E-14, -46.66904755831211560, 85.00100000000000477 ) ) ;
#6536=CARTESIAN_POINT ( 'NONE',  ( -20.55634918610408945, -31.11269837220804035, 0.000000000000000000 ) ) ;
#6560=DIRECTION ( 'NONE',  ( -0.000000000000000000, -0.000000000000000000, -1.000000000000000000 ) ) ;
#6573=PLANE ( 'NONE',  #21847 ) ;
#6591=AXIS2_PLACEMENT_3D ( 'NONE', #32062, #49259, #21492 ) ;
#6600=ORIENTED_EDGE ( 'NONE', *, *, #51176, .T. ) ;
#6604=FACE_OUTER_BOUND ( 'NONE', #60316, .T. ) ;
#6635=PLANE ( 'NONE',  #50738 ) ;
#6641=EDGE_LOOP ( 'NONE', ( #22876, #55136, #43742, #23512 ) ) ;
#6643=CARTESIAN_POINT ( 'NONE',  ( -5.000000000000000000, 0.000000000000000000, 2.000000000000001776 ) ) ;
#6661=DIRECTION ( 'NONE',  ( 0.000000000000000000, 1.000000000000000000, -0.000000000000000000 ) ) ;
#6665=ORIENTED_EDGE ( 'NONE', *, *, #33922, .F. ) ;
#6676=ADVANCED_FACE ( 'NONE', ( #24511 ), #56856, .T. ) ;
#6678=ORIENTED_EDGE ( 'NONE', *, *, #37088, .T. ) ;
#6689=LINE ( 'NONE', #25571, #26039 ) ;
#6724=CARTESIAN_POINT ( 'NONE',  ( 15.55634918610411610, 51.66904755831205875, 2.000000000000001776 ) ) ;
#6738=VERTEX_POINT ( 'NONE', #22012 ) ;
#6751=DIRECTION ( 'NONE',  ( -1.000000000000000000, 0.000000000000000000, 0.000000000000000000 ) ) ;
#6753=CARTESIAN_POINT ( 'NONE',  ( -51.66904755831212981, -15.55634918610397222, 85.00100000000000477 ) ) ;
#6766=EDGE_CURVE ( 'NONE', #41218, #23252, #59978, .T. ) ;
#6781=LINE ( 'NONE', #22968, #54070 ) ;
#6788=CARTESIAN_POINT ( 'NONE',  ( -31.11269837220809364, -10.55634918610397932, 0.000000000000000000 ) ) ;
#6809=ORIENTED_EDGE ( 'NONE', *, *, #6511, .F. ) ;
#6813=VECTOR ( 'NONE', #11142, 1000.000000000000000 ) ;
#6861=CARTESIAN_POINT ( 'NONE',  ( -20.55634918610403261, 2.818925648462311528E-14, 85.00100000000000477 ) ) ;
#6897=VECTOR ( 'NONE', #42343, 1000.000000000000000 ) ;
#6951=CARTESIAN_POINT ( 'NONE',  ( -4.999999999999936939, 31.11269837220806167, 2.000000000000001776 ) ) ;
#6952=ORIENTED_EDGE ( 'NONE', *, *, #12726, .F. ) ;
#6964=DIRECTION ( 'NONE',  ( 1.000000000000000000, 0.000000000000000000, 0.000000000000000000 ) ) ;
#6976=ORIENTED_EDGE ( 'NONE', *, *, #57804, .T. ) ;
#6983=CARTESIAN_POINT ( 'NONE',  ( -31.11269837220804035, 15.55634918610408945, 85.00100000000000477 ) ) ;
#7009=CARTESIAN_POINT ( 'NONE',  ( 26.11269837220806167, -6.375108774214766072E-14, 85.00100000000000477 ) ) ;
#7021=CARTESIAN_POINT ( 'NONE',  ( -31.11269837220801193, 31.11269837220812207, 2.000000000000001776 ) ) ;
#7055=VECTOR ( 'NONE', #11401, 1000.000000000000000 ) ;
#7060=LINE ( 'NONE', #59811, #35527 ) ;
#7079=ADVANCED_FACE ( 'NONE', ( #21573 ), #11361, .F. ) ;
#7084=CARTESIAN_POINT ( 'NONE',  ( 15.55634918610409656, 31.11269837220803325, 2.000000000000001776 ) ) ;
#7085=DIRECTION ( 'NONE',  ( -1.000000000000000000, 0.000000000000000000, 0.000000000000000000 ) ) ;
#7094=AXIS2_PLACEMENT_3D ( 'NONE', #23196, #17913, #53178 ) ;
#7106=AXIS2_PLACEMENT_3D ( 'NONE', #61590, #12706, #13064 ) ;
#7128=VERTEX_POINT ( 'NONE', #21920 ) ;
#7143=CARTESIAN_POINT ( 'NONE',  ( -15.55634918610408945, -26.11269837220804035, 85.00100000000000477 ) ) ;
#7156=VECTOR ( 'NONE', #24769, 1000.000000000000000 ) ;
#7157=DIRECTION ( 'NONE',  ( 0.000000000000000000, 1.000000000000000000, 0.000000000000000000 ) ) ;
#7162=DIRECTION ( 'NONE',  ( -0.000000000000000000, -0.000000000000000000, -1.000000000000000000 ) ) ;
#7175=ORIENTED_EDGE ( 'NONE', *, *, #69066, .F. ) ;
#7177=ORIENTED_EDGE ( 'NONE', *, *, #28666, .T. ) ;
#7178=CARTESIAN_POINT ( 'NONE',  ( 15.55634918610397399, -31.11269837220809364, 0.000000000000000000 ) ) ;
#7206=AXIS2_PLACEMENT_3D ( 'NONE', #32689, #60109, #28101 ) ;
#7215=CARTESIAN_POINT ( 'NONE',  ( 10.55634918610400419, -10.55634918610406281, 0.000000000000000000 ) ) ;
#7216=ORIENTED_EDGE ( 'NONE', *, *, #52976, .T. ) ;
#7221=CARTESIAN_POINT ( 'NONE',  ( 26.11269837220812562, 31.11269837220800483, 0.000000000000000000 ) ) ;
#7227=DIRECTION ( 'NONE',  ( 0.000000000000000000, -1.000000000000000000, 0.000000000000000000 ) ) ;
#7264=ORIENTED_EDGE ( 'NONE', *, *, #62105, .F. ) ;
#7271=CARTESIAN_POINT ( 'NONE',  ( 46.66904755831212981, 15.55634918610394379, 0.000000000000000000 ) ) ;
#7302=DIRECTION ( 'NONE',  ( 0.000000000000000000, 1.000000000000000000, -0.000000000000000000 ) ) ;
#7311=ADVANCED_FACE ( 'NONE', ( #16563 ), #6241, .F. ) ;
#7323=DIRECTION ( 'NONE',  ( -1.000000000000000000, 0.000000000000000000, 0.000000000000000000 ) ) ;
#7325=FACE_BOUND ( 'NONE', #65276, .T. ) ;
#7332=EDGE_LOOP ( 'NONE', ( #29634, #1904, #39614, #32845 ) ) ;
#7335=DIRECTION ( 'NONE',  ( -0.000000000000000000, -0.000000000000000000, -1.000000000000000000 ) ) ;
#7347=EDGE_LOOP ( 'NONE', ( #15337, #14138, #8915, #52146 ) ) ;
#7401=ADVANCED_FACE ( 'NONE', ( #39082 ), #33796, .F. ) ;
#7405=CARTESIAN_POINT ( 'NONE',  ( 15.55634918610411610, 51.66904755831205875, 85.00100000000000477 ) ) ;
#7410=ORIENTED_EDGE ( 'NONE', *, *, #12813, .T. ) ;
#7425=EDGE_LOOP ( 'NONE', ( #6600, #59641, #25600, #28610 ) ) ;
#7450=ORIENTED_EDGE ( 'NONE', *, *, #20809, .T. ) ;
#7458=DIRECTION ( 'NONE',  ( 1.000000000000000000, -0.000000000000000000, -0.000000000000000000 ) ) ;
#7489=CARTESIAN_POINT ( 'NONE',  ( -20.55634918610396866, 36.11269837220808654, 85.00100000000000477 ) ) ;
#7492=ORIENTED_EDGE ( 'NONE', *, *, #1164, .F. ) ;
#7527=VERTEX_POINT ( 'NONE', #33287 ) ;
#7552=DIRECTION ( 'NONE',  ( 0.000000000000000000, 0.000000000000000000, -1.000000000000000000 ) ) ;
#7568=AXIS2_PLACEMENT_3D ( 'NONE', #42209, #4570, #4237 ) ;
#7572=VERTEX_POINT ( 'NONE', #17800 ) ;
#7607=AXIS2_PLACEMENT_3D ( 'NONE', #45506, #54043, #11486 ) ;
#7617=FACE_OUTER_BOUND ( 'NONE', #49306, .T. ) ;
#7661=EDGE_CURVE ( 'NONE', #16146, #17510, #62442, .T. ) ;
#7662=EDGE_CURVE ( 'NONE', #34612, #36801, #57508, .T. ) ;
#7676=FACE_BOUND ( 'NONE', #25045, .T. ) ;
#7679=LINE ( 'NONE', #51281, #67959 ) ;
#7694=ORIENTED_EDGE ( 'NONE', *, *, #26148, .T. ) ;
#7710=CARTESIAN_POINT ( 'NONE',  ( 7.762887554996211747E-14, 51.66904755831208718, 85.00100000000000477 ) ) ;
#7717=FACE_OUTER_BOUND ( 'NONE', #45172, .T. ) ;
#7727=DIRECTION ( 'NONE',  ( -1.000000000000000000, 0.000000000000000000, 0.000000000000000000 ) ) ;
#7740=EDGE_CURVE ( 'NONE', #67838, #11106, #32839, .T. ) ;
#7751=EDGE_LOOP ( 'NONE', ( #37065, #32453, #22846, #15459 ) ) ;
#7767=DIRECTION ( 'NONE',  ( 1.000000000000000000, -0.000000000000000000, -0.000000000000000000 ) ) ;
#7791=ORIENTED_EDGE ( 'NONE', *, *, #54955, .F. ) ;
#7796=CARTESIAN_POINT ( 'NONE',  ( -36.11269837220806522, 5.594483210025202879E-14, 2.000000000000001776 ) ) ;
#7803=ORIENTED_EDGE ( 'NONE', *, *, #49798, .T. ) ;
#7814=CARTESIAN_POINT ( 'NONE',  ( 74.99999999999998579, 0.000000000000000000, 25.00000000000007816 ) ) ;
#7843=VECTOR ( 'NONE', #52125, 1000.000000000000000 ) ;
#7850=ORIENTED_EDGE ( 'NONE', *, *, #19845, .F. ) ;
#7864=ORIENTED_EDGE ( 'NONE', *, *, #36472, .T. ) ;
#7874=ORIENTED_EDGE ( 'NONE', *, *, #48965, .T. ) ;
#7943=EDGE_CURVE ( 'NONE', #26420, #56407, #39177, .T. ) ;
#7950=LINE ( 'NONE', #29402, #36235 ) ;
#7959=LINE ( 'NONE', #38569, #15229 ) ;
#7962=VECTOR ( 'NONE', #11060, 1000.000000000000000 ) ;
#7985=LINE ( 'NONE', #19220, #15675 ) ;
#7988=EDGE_LOOP ( 'NONE', ( #45962, #24395 ) ) ;
#7989=CARTESIAN_POINT ( 'NONE',  ( -36.11269837220812207, -31.11269837220801193, 85.00100000000000477 ) ) ;
#8007=FACE_BOUND ( 'NONE', #31326, .T. ) ;
#8029=ORIENTED_EDGE ( 'NONE', *, *, #37873, .F. ) ;
#8039=DIRECTION ( 'NONE',  ( -0.000000000000000000, -0.000000000000000000, 1.000000000000000000 ) ) ;
#8051=LINE ( 'NONE', #44987, #53562 ) ;
#8056=ORIENTED_EDGE ( 'NONE', *, *, #22313, .F. ) ;
#8108=CARTESIAN_POINT ( 'NONE',  ( 0.000000000000000000, 0.000000000000000000, 2.000000000000001776 ) ) ;
#8115=VECTOR ( 'NONE', #52378, 1000.000000000000000 ) ;
#8128=VECTOR ( 'NONE', #59536, 1000.000000000000000 ) ;
#8182=CARTESIAN_POINT ( 'NONE',  ( -31.11269837220801193, 36.11269837220812207, 2.000000000000001776 ) ) ;
#8204=VECTOR ( 'NONE', #24155, 1000.000000000000000 ) ;
#8206=ORIENTED_EDGE ( 'NONE', *, *, #23233, .F. ) ;
#8213=ADVANCED_FACE ( 'NONE', ( #40129 ), #61586, .F. ) ;
#8218=ADVANCED_FACE ( 'NONE', ( #36924 ), #53075, .F. ) ;
#8228=FACE_OUTER_BOUND ( 'NONE', #21228, .T. ) ;
#8235=FACE_OUTER_BOUND ( 'NONE', #56113, .T. ) ;
#8237=CARTESIAN_POINT ( 'NONE',  ( -15.55634918610396866, 36.11269837220808654, 0.000000000000000000 ) ) ;
#8255=DIRECTION ( 'NONE',  ( 0.000000000000000000, -0.000000000000000000, -1.000000000000000000 ) ) ;
#8273=DIRECTION ( 'NONE',  ( 0.000000000000000000, 1.000000000000000000, 0.000000000000000000 ) ) ;
#8281=AXIS2_PLACEMENT_3D ( 'NONE', #36421, #55892, #57877 ) ;
#8293=VERTEX_POINT ( 'NONE', #9850 ) ;
#8308=CARTESIAN_POINT ( 'NONE',  ( -46.66904755831210139, 5.000000000000066613, 85.00100000000000477 ) ) ;
#8316=VECTOR ( 'NONE', #13758, 1000.000000000000000 ) ;
#8319=DIRECTION ( 'NONE',  ( 1.000000000000000000, 0.000000000000000000, 0.000000000000000000 ) ) ;
#8325=DIRECTION ( 'NONE',  ( 1.000000000000000000, -0.000000000000000000, -0.000000000000000000 ) ) ;
#8329=VECTOR ( 'NONE', #54065, 1000.000000000000000 ) ;
#8344=ADVANCED_FACE ( 'NONE', ( #41858 ), #47457, .F. ) ;
#8348=CARTESIAN_POINT ( 'NONE',  ( -2.645453300864630819E-14, -15.55634918610403616, 0.000000000000000000 ) ) ;
#8368=EDGE_LOOP ( 'NONE', ( #29024, #5978, #40048, #32895 ) ) ;
#8416=VERTEX_POINT ( 'NONE', #18238 ) ;
#8422=AXIS2_PLACEMENT_3D ( 'NONE', #51604, #13617, #19942 ) ;
#8433=DIRECTION ( 'NONE',  ( -1.000000000000000000, 0.000000000000000000, 0.000000000000000000 ) ) ;
#8469=CARTESIAN_POINT ( 'NONE',  ( 31.11269837220803325, -10.55634918610409656, 85.00100000000000477 ) ) ;
#8482=ORIENTED_EDGE ( 'NONE', *, *, #24944, .T. ) ;
#8489=CARTESIAN_POINT ( 'NONE',  ( -5.767955557622883589E-14, -26.11269837220806522, 0.000000000000000000 ) ) ;
#8493=CARTESIAN_POINT ( 'NONE',  ( 26.11269837220812562, 31.11269837220800483, 0.000000000000000000 ) ) ;
#8504=VERTEX_POINT ( 'NONE', #67475 ) ;
#8516=VERTEX_POINT ( 'NONE', #19270 ) ;
#8521=CARTESIAN_POINT ( 'NONE',  ( 15.55634918610409656, 31.11269837220803325, 85.00100000000000477 ) ) ;
#8531=DIRECTION ( 'NONE',  ( 0.000000000000000000, 0.000000000000000000, -1.000000000000000000 ) ) ;
#8539=FACE_OUTER_BOUND ( 'NONE', #65335, .T. ) ;
#8542=VERTEX_POINT ( 'NONE', #4819 ) ;
#8552=PLANE ( 'NONE',  #16277 ) ;
#8568=DIRECTION ( 'NONE',  ( 1.000000000000000000, -0.000000000000000000, -0.000000000000000000 ) ) ;
#8574=ORIENTED_EDGE ( 'NONE', *, *, #62429, .T. ) ;
#8586=CARTESIAN_POINT ( 'NONE',  ( -31.11269837220804035, 20.55634918610408945, 85.00100000000000477 ) ) ;
#8597=LINE ( 'NONE', #18102, #65289 ) ;
#8601=DIRECTION ( 'NONE',  ( 1.000000000000000000, 0.000000000000000000, 0.000000000000000000 ) ) ;
#8605=VERTEX_POINT ( 'NONE', #65305 ) ;
#8613=VECTOR ( 'NONE', #3544, 1000.000000000000000 ) ;
#8688=ORIENTED_EDGE ( 'NONE', *, *, #63155, .T. ) ;
#8716=VECTOR ( 'NONE', #61722, 1000.000000000000000 ) ;
#8720=VECTOR ( 'NONE', #64952, 1000.000000000000000 ) ;
#8741=ORIENTED_EDGE ( 'NONE', *, *, #49210, .F. ) ;
#8745=VERTEX_POINT ( 'NONE', #42295 ) ;
#8755=ORIENTED_EDGE ( 'NONE', *, *, #26991, .F. ) ;
#8773=VECTOR ( 'NONE', #60600, 1000.000000000000000 ) ;
#8788=ORIENTED_EDGE ( 'NONE', *, *, #1909, .T. ) ;
#8798=ORIENTED_EDGE ( 'NONE', *, *, #54860, .T. ) ;
#8807=ORIENTED_EDGE ( 'NONE', *, *, #38183, .T. ) ;
#8812=EDGE_CURVE ( 'NONE', #13372, #64405, #2168, .T. ) ;
#8816=LINE ( 'NONE', #47118, #43368 ) ;
#8825=EDGE_CURVE ( 'NONE', #5765, #47170, #55617, .T. ) ;
#8862=VECTOR ( 'NONE', #2836, 1000.000000000000000 ) ;
#8886=ORIENTED_EDGE ( 'NONE', *, *, #51955, .F. ) ;
#8915=ORIENTED_EDGE ( 'NONE', *, *, #39313, .F. ) ;
#8941=DIRECTION ( 'NONE',  ( 1.000000000000000000, -0.000000000000000000, -0.000000000000000000 ) ) ;
#8949=DIRECTION ( 'NONE',  ( 0.000000000000000000, 0.000000000000000000, 1.000000000000000000 ) ) ;
#8951=ORIENTED_EDGE ( 'NONE', *, *, #3648, .F. ) ;
#8952=PLANE ( 'NONE',  #21090 ) ;
#8963=EDGE_CURVE ( 'NONE', #52465, #37055, #66205, .T. ) ;
#8967=DIRECTION ( 'NONE',  ( 0.000000000000000000, 1.000000000000000000, -0.000000000000000000 ) ) ;
#8974=DIRECTION ( 'NONE',  ( 0.000000000000000000, 1.000000000000000000, -0.000000000000000000 ) ) ;
#8975=CARTESIAN_POINT ( 'NONE',  ( -4.999999999999922728, 51.66904755831208718, 2.000000000000001776 ) ) ;
#8977=EDGE_CURVE ( 'NONE', #13387, #65364, #57015, .T. ) ;
#8981=LINE ( 'NONE', #30429, #43221 ) ;
#8987=ADVANCED_FACE ( 'NONE', ( #56661 ), #46441, .F. ) ;
#8994=DIRECTION ( 'NONE',  ( 0.000000000000000000, -1.000000000000000000, 0.000000000000000000 ) ) ;
#9001=DIRECTION ( 'NONE',  ( 0.000000000000000000, -1.000000000000000000, 0.000000000000000000 ) ) ;
#9023=PRODUCT_CONTEXT ( 'NONE', #45341, 'mechanical' ) ;
#9025=CARTESIAN_POINT ( 'NONE',  ( -36.11269837220809364, -15.55634918610397754, 2.000000000000000000 ) ) ;
#9039=VECTOR ( 'NONE', #68090, 1000.000000000000000 ) ;
#9041=LINE ( 'NONE', #35424, #38372 ) ;
#9042=CARTESIAN_POINT ( 'NONE',  ( 26.11269837220812562, 36.11269837220800838, 0.000000000000000000 ) ) ;
#9053=FACE_BOUND ( 'NONE', #5303, .T. ) ;
#9078=VECTOR ( 'NONE', #44320, 1000.000000000000000 ) ;
#9089=DIRECTION ( 'NONE',  ( 1.000000000000000000, -0.000000000000000000, 0.000000000000000000 ) ) ;
#9109=DIRECTION ( 'NONE',  ( -0.000000000000000000, -0.000000000000000000, -1.000000000000000000 ) ) ;
#9130=CARTESIAN_POINT ( 'NONE',  ( 15.55634918610406103, 15.55634918610400241, 0.000000000000000000 ) ) ;
#9159=CARTESIAN_POINT ( 'NONE',  ( 6.375108774214766072E-14, 36.11269837220805812, 2.000000000000001776 ) ) ;
#9169=DIRECTION ( 'NONE',  ( -0.000000000000000000, -0.000000000000000000, -1.000000000000000000 ) ) ;
#9180=CARTESIAN_POINT ( 'NONE',  ( -20.55634918610411077, -46.66904755831208718, 2.000000000000000000 ) ) ;
#9183=ORIENTED_EDGE ( 'NONE', *, *, #41454, .T. ) ;
#9200=EDGE_CURVE ( 'NONE', #30237, #57581, #39022, .T. ) ;
#9205=DIRECTION ( 'NONE',  ( 1.000000000000000000, -0.000000000000000000, -0.000000000000000000 ) ) ;
#9216=AXIS2_PLACEMENT_3D ( 'NONE', #56295, #56647, #55248 ) ;
#9260=PLANE ( 'NONE',  #31759 ) ;
#9264=CARTESIAN_POINT ( 'NONE',  ( -36.11269837220804391, 15.55634918610408945, 0.000000000000000000 ) ) ;
#9274=CARTESIAN_POINT ( 'NONE',  ( 15.55634918610403261, 0.000000000000000000, 0.000000000000000000 ) ) ;
#9284=ORIENTED_EDGE ( 'NONE', *, *, #57336, .F. ) ;
#9290=LINE ( 'NONE', #57144, #63732 ) ;
#9306=ORIENTED_EDGE ( 'NONE', *, *, #28463, .F. ) ;
#9324=CARTESIAN_POINT ( 'NONE',  ( 10.55634918610406281, 15.55634918610400241, 85.00100000000000477 ) ) ;
#9331=CARTESIAN_POINT ( 'NONE',  ( -5.000000000000073719, -46.66904755831211560, 85.00100000000000477 ) ) ;
#9332=ORIENTED_EDGE ( 'NONE', *, *, #20722, .F. ) ;
#9340=DIRECTION ( 'NONE',  ( 0.000000000000000000, 0.000000000000000000, 1.000000000000000000 ) ) ;
#9365=EDGE_LOOP ( 'NONE', ( #28126, #1997, #15700, #68418 ) ) ;
#9366=VECTOR ( 'NONE', #7323, 1000.000000000000000 ) ;
#9370=PLANE ( 'NONE',  #40593 ) ;
#9384=ORIENTED_EDGE ( 'NONE', *, *, #37296, .F. ) ;
#9398=DIRECTION ( 'NONE',  ( 0.000000000000000000, 0.000000000000000000, 1.000000000000000000 ) ) ;
#9428=DIRECTION ( 'NONE',  ( -1.000000000000000000, 0.000000000000000000, 0.000000000000000000 ) ) ;
#9437=EDGE_LOOP ( 'NONE', ( #3244, #21939, #10507, #34679 ) ) ;
#9438=DIRECTION ( 'NONE',  ( 1.000000000000000000, -0.000000000000000000, -0.000000000000000000 ) ) ;
#9458=AXIS2_PLACEMENT_3D ( 'NONE', #56331, #17664, #34554 ) ;
#9469=VECTOR ( 'NONE', #5942, 1000.000000000000000 ) ;
#9479=DIRECTION ( 'NONE',  ( -1.000000000000000000, 0.000000000000000000, 0.000000000000000000 ) ) ;
#9494=ORIENTED_EDGE ( 'NONE', *, *, #63914, .F. ) ;
#9519=ORIENTED_EDGE ( 'NONE', *, *, #51386, .F. ) ;
#9550=ORIENTED_EDGE ( 'NONE', *, *, #39019, .F. ) ;
#9575=CARTESIAN_POINT ( 'NONE',  ( -51.66904755831210139, 6.635317295611287136E-14, 85.00100000000000477 ) ) ;
#9589=ORIENTED_EDGE ( 'NONE', *, *, #36903, .F. ) ;
#9597=EDGE_CURVE ( 'NONE', #41430, #19049, #287, .T. ) ;
#9604=ORIENTED_EDGE ( 'NONE', *, *, #23572, .T. ) ;
#9611=CARTESIAN_POINT ( 'NONE',  ( 66.50000000000000000, 0.000000000000000000, -0.002000000000002000178 ) ) ;
#9618=PLANE ( 'NONE',  #306 ) ;
#9642=CARTESIAN_POINT ( 'NONE',  ( 10.55634918610411432, 51.66904755831205875, 2.000000000000001776 ) ) ;
#9664=ORIENTED_EDGE ( 'NONE', *, *, #18763, .F. ) ;
#9686=ORIENTED_EDGE ( 'NONE', *, *, #34175, .T. ) ;
#9695=DIRECTION ( 'NONE',  ( 0.000000000000000000, 1.000000000000000000, -0.000000000000000000 ) ) ;
#9723=VECTOR ( 'NONE', #7085, 1000.000000000000000 ) ;
#9743=DIRECTION ( 'NONE',  ( 0.000000000000000000, 0.000000000000000000, 1.000000000000000000 ) ) ;
#9781=PLANE ( 'NONE',  #51094 ) ;
#9803=VECTOR ( 'NONE', #1853, 1000.000000000000000 ) ;
#9833=CARTESIAN_POINT ( 'NONE',  ( -20.55634918610400419, 15.55634918610405748, 0.000000000000000000 ) ) ;
#9844=CARTESIAN_POINT ( 'NONE',  ( 15.55634918610406103, 20.55634918610400064, 85.00100000000000477 ) ) ;
#9850=CARTESIAN_POINT ( 'NONE',  ( 46.66904755831210139, 4.999999999999909406, 0.000000000000000000 ) ) ;
#9860=DIRECTION ( 'NONE',  ( 0.000000000000000000, 0.000000000000000000, -1.000000000000000000 ) ) ;
#9863=ADVANCED_FACE ( 'NONE', ( #21667 ), #42768, .F. ) ;
#9910=ORIENTED_EDGE ( 'NONE', *, *, #43805, .F. ) ;
#9924=CARTESIAN_POINT ( 'NONE',  ( 31.11269837220803325, -15.55634918610409656, 0.000000000000000000 ) ) ;
#9946=LINE ( 'NONE', #56481, #54324 ) ;
#9948=ORIENTED_EDGE ( 'NONE', *, *, #20809, .F. ) ;
#9953=CARTESIAN_POINT ( 'NONE',  ( -7.329206686002009974E-14, -46.66904755831211560, 2.000000000000001776 ) ) ;
#9960=CARTESIAN_POINT ( 'NONE',  ( 15.55634918610397399, -31.11269837220809364, 2.000000000000001776 ) ) ;
#9968=VERTEX_POINT ( 'NONE', #19169 ) ;
#9997=CYLINDRICAL_SURFACE ( 'NONE', #58334, 74.99999999999998579 ) ;
#10001=VECTOR ( 'NONE', #51518, 1000.000000000000000 ) ;
#10009=DIRECTION ( 'NONE',  ( -1.000000000000000000, 0.000000000000000000, 0.000000000000000000 ) ) ;
#10031=PLANE ( 'NONE',  #33315 ) ;
#10034=ORIENTED_EDGE ( 'NONE', *, *, #14314, .T. ) ;
#10038=CARTESIAN_POINT ( 'NONE',  ( 0.000000000000000000, 5.000000000000000000, 85.00100000000000477 ) ) ;
#10077=DIRECTION ( 'NONE',  ( -0.000000000000000000, -0.000000000000000000, -1.000000000000000000 ) ) ;
#10085=DIRECTION ( 'NONE',  ( -0.000000000000000000, -0.000000000000000000, -1.000000000000000000 ) ) ;
#10140=CARTESIAN_POINT ( 'NONE',  ( 31.11269837220803325, -10.55634918610409656, 2.000000000000001776 ) ) ;
#10166=ORIENTED_EDGE ( 'NONE', *, *, #45081, .T. ) ;
#10168=VERTEX_POINT ( 'NONE', #8975 ) ;
#10176=CARTESIAN_POINT ( 'NONE',  ( -7.329206686002009974E-14, -46.66904755831211560, 2.000000000000001776 ) ) ;
#10196=DIRECTION ( 'NONE',  ( 0.000000000000000000, -0.000000000000000000, -1.000000000000000000 ) ) ;
#10200=VERTEX_POINT ( 'NONE', #1177 ) ;
#10230=EDGE_CURVE ( 'NONE', #30657, #34238, #59209, .T. ) ;
#10259=AXIS2_PLACEMENT_3D ( 'NONE', #19459, #40566, #30024 ) ;
#10273=CARTESIAN_POINT ( 'NONE',  ( 15.55634918610406103, 20.55634918610400064, 0.000000000000000000 ) ) ;
#10276=ORIENTED_EDGE ( 'NONE', *, *, #39806, .T. ) ;
#10290=EDGE_CURVE ( 'NONE', #33258, #57934, #48293, .T. ) ;
#10303=ADVANCED_FACE ( 'NONE', ( #64503 ), #10337, .F. ) ;
#10307=VECTOR ( 'NONE', #68733, 1000.000000000000000 ) ;
#10337=PLANE ( 'NONE',  #3094 ) ;
#10348=VECTOR ( 'NONE', #67867, 1000.000000000000000 ) ;
#10376=VERTEX_POINT ( 'NONE', #50413 ) ;
#10394=ADVANCED_FACE ( 'NONE', ( #20462 ), #3267, .F. ) ;
#10395=LINE ( 'NONE', #42752, #37523 ) ;
#10400=VECTOR ( 'NONE', #16824, 1000.000000000000000 ) ;
#10408=FACE_BOUND ( 'NONE', #13332, .T. ) ;
#10442=CARTESIAN_POINT ( 'NONE',  ( -20.55634918610403261, 5.000000000000028422, 0.000000000000000000 ) ) ;
#10449=LINE ( 'NONE', #22398, #6813 ) ;
#10474=LINE ( 'NONE', #59353, #4177 ) ;
#10487=LINE ( 'NONE', #48111, #65366 ) ;
#10507=ORIENTED_EDGE ( 'NONE', *, *, #36534, .F. ) ;
#10544=ADVANCED_FACE ( 'NONE', ( #3603 ), #25071, .F. ) ;
#10556=DIRECTION ( 'NONE',  ( 0.000000000000000000, 0.000000000000000000, 1.000000000000000000 ) ) ;
#10571=ORIENTED_EDGE ( 'NONE', *, *, #60873, .F. ) ;
#10574=ORIENTED_EDGE ( 'NONE', *, *, #58374, .F. ) ;
#10578=ORIENTED_EDGE ( 'NONE', *, *, #5300, .T. ) ;
#10624=ADVANCED_FACE ( 'NONE', ( #54543 ), #48214, .F. ) ;
#10630=FACE_OUTER_BOUND ( 'NONE', #20860, .T. ) ;
#10640=VECTOR ( 'NONE', #51083, 1000.000000000000000 ) ;
#10647=VECTOR ( 'NONE', #52928, 1000.000000000000000 ) ;
#10664=VERTEX_POINT ( 'NONE', #16569 ) ;
#10678=DIRECTION ( 'NONE',  ( -0.000000000000000000, -0.000000000000000000, -1.000000000000000000 ) ) ;
#10703=ORIENTED_EDGE ( 'NONE', *, *, #56157, .T. ) ;
#10708=ADVANCED_FACE ( 'NONE', ( #45042 ), #57251, .F. ) ;
#10709=DIRECTION ( 'NONE',  ( 1.000000000000000000, -0.000000000000000000, 0.000000000000000000 ) ) ;
#10716=CARTESIAN_POINT ( 'NONE',  ( 6.375108774214766072E-14, 36.11269837220805812, 2.000000000000001776 ) ) ;
#10728=EDGE_CURVE ( 'NONE', #11517, #64911, #17260, .T. ) ;
#10770=DIRECTION ( 'NONE',  ( -1.000000000000000000, 0.000000000000000000, 0.000000000000000000 ) ) ;
#10804=EDGE_LOOP ( 'NONE', ( #48687, #23451, #50641, #18575 ) ) ;
#10808=DIRECTION ( 'NONE',  ( 0.000000000000000000, -1.000000000000000000, 0.000000000000000000 ) ) ;
#10846=DIRECTION ( 'NONE',  ( 0.000000000000000000, 0.000000000000000000, -1.000000000000000000 ) ) ;
#10859=EDGE_LOOP ( 'NONE', ( #40307, #14428, #62803, #55921 ) ) ;
#10872=EDGE_CURVE ( 'NONE', #38069, #32692, #41422, .T. ) ;
#10897=CARTESIAN_POINT ( 'NONE',  ( -20.55634918610408945, -26.11269837220804035, 0.000000000000000000 ) ) ;
#10912=VERTEX_POINT ( 'NONE', #31898 ) ;
#10927=VECTOR ( 'NONE', #60724, 1000.000000000000000 ) ;
#10932=DIRECTION ( 'NONE',  ( -1.000000000000000000, 0.000000000000000000, 0.000000000000000000 ) ) ;
#10970=VERTEX_POINT ( 'NONE', #27649 ) ;
#10975=LINE ( 'NONE', #25797, #56619 ) ;
#10989=VECTOR ( 'NONE', #60744, 1000.000000000000000 ) ;
#11024=ORIENTED_EDGE ( 'NONE', *, *, #58374, .T. ) ;
#11037=DIRECTION ( 'NONE',  ( -1.000000000000000000, 0.000000000000000000, 0.000000000000000000 ) ) ;
#11058=VERTEX_POINT ( 'NONE', #17811 ) ;
#11060=DIRECTION ( 'NONE',  ( 0.000000000000000000, 1.000000000000000000, 0.000000000000000000 ) ) ;
#11069=CARTESIAN_POINT ( 'NONE',  ( -31.11269837220801193, 36.11269837220812207, 0.000000000000000000 ) ) ;
#11076=EDGE_CURVE ( 'NONE', #60572, #10912, #5842, .T. ) ;
#11089=VECTOR ( 'NONE', #49055, 1000.000000000000000 ) ;
#11098=EDGE_CURVE ( 'NONE', #31799, #51103, #12183, .T. ) ;
#11106=VERTEX_POINT ( 'NONE', #49794 ) ;
#11109=ORIENTED_EDGE ( 'NONE', *, *, #4123, .F. ) ;
#11131=LINE ( 'NONE', #54020, #35184 ) ;
#11139=LINE ( 'NONE', #32604, #5179 ) ;
#11142=DIRECTION ( 'NONE',  ( -0.000000000000000000, -0.000000000000000000, -1.000000000000000000 ) ) ;
#11143=VECTOR ( 'NONE', #50892, 1000.000000000000000 ) ;
#11151=CARTESIAN_POINT ( 'NONE',  ( -15.55634918610408945, -26.11269837220804035, 0.000000000000000000 ) ) ;
#11163=VERTEX_POINT ( 'NONE', #50158 ) ;
#11180=LINE ( 'NONE', #22092, #48397 ) ;
#11192=CARTESIAN_POINT ( 'NONE',  ( 15.55634918610400241, -10.55634918610406281, 0.000000000000000000 ) ) ;
#11208=ORIENTED_EDGE ( 'NONE', *, *, #8825, .F. ) ;
#11222=VERTEX_POINT ( 'NONE', #51555 ) ;
#11223=PLANE ( 'NONE',  #17333 ) ;
#11233=ORIENTED_EDGE ( 'NONE', *, *, #56157, .F. ) ;
#11245=EDGE_CURVE ( 'NONE', #55744, #30631, #39607, .T. ) ;
#11258=EDGE_LOOP ( 'NONE', ( #59654, #69321, #293, #21113 ) ) ;
#11265=VECTOR ( 'NONE', #67403, 1000.000000000000000 ) ;
#11279=ORIENTED_EDGE ( 'NONE', *, *, #23203, .T. ) ;
#11298=CARTESIAN_POINT ( 'NONE',  ( 31.11269837220806522, 4.999999999999936939, 2.000000000000001776 ) ) ;
#11299=CARTESIAN_POINT ( 'NONE',  ( -36.11269837220806522, 5.594483210025202879E-14, 85.00100000000000477 ) ) ;
#11300=VECTOR ( 'NONE', #3043, 1000.000000000000000 ) ;
#11310=VECTOR ( 'NONE', #906, 1000.000000000000000 ) ;
#11316=ORIENTED_EDGE ( 'NONE', *, *, #46935, .T. ) ;
#11322=CARTESIAN_POINT ( 'NONE',  ( -15.55634918610405748, -15.55634918610400774, 2.000000000000001776 ) ) ;
#11325=LINE ( 'NONE', #58148, #47506 ) ;
#11330=LINE ( 'NONE', #43340, #958 ) ;
#11340=ORIENTED_EDGE ( 'NONE', *, *, #51826, .T. ) ;
#11361=PLANE ( 'NONE',  #55610 ) ;
#11362=CARTESIAN_POINT ( 'NONE',  ( 15.55634918610409656, 31.11269837220803325, 85.00100000000000477 ) ) ;
#11365=AXIS2_PLACEMENT_3D ( 'NONE', #47209, #14859, #20478 ) ;
#11375=EDGE_LOOP ( 'NONE', ( #16067, #20445, #32376, #28073 ) ) ;
#11377=ORIENTED_EDGE ( 'NONE', *, *, #26096, .T. ) ;
#11379=LINE ( 'NONE', #60283, #27564 ) ;
#11394=ORIENTED_EDGE ( 'NONE', *, *, #59630, .F. ) ;
#11401=DIRECTION ( 'NONE',  ( -0.000000000000000000, -0.000000000000000000, -1.000000000000000000 ) ) ;
#11407=AXIS2_PLACEMENT_3D ( 'NONE', #49219, #58735, #10556 ) ;
#11416=ORIENTED_EDGE ( 'NONE', *, *, #59692, .T. ) ;
#11433=VERTEX_POINT ( 'NONE', #19803 ) ;
#11435=FACE_BOUND ( 'NONE', #39026, .T. ) ;
#11441=AXIS2_PLACEMENT_3D ( 'NONE', #66148, #1764, #17586 ) ;
#11457=AXIS2_PLACEMENT_3D ( 'NONE', #64665, #48804, #6964 ) ;
#11459=AXIS2_PLACEMENT_3D ( 'NONE', #28055, #65006, #65353 ) ;
#11484=FACE_OUTER_BOUND ( 'NONE', #40433, .T. ) ;
#11486=DIRECTION ( 'NONE',  ( 1.000000000000000000, 0.000000000000000000, 0.000000000000000000 ) ) ;
#11490=ORIENTED_EDGE ( 'NONE', *, *, #64711, .F. ) ;
#11495=LINE ( 'NONE', #38242, #10989 ) ;
#11507=EDGE_LOOP ( 'NONE', ( #3646, #35535, #17041, #24530 ) ) ;
#11508=CARTESIAN_POINT ( 'NONE',  ( -15.55634918610403439, 2.818925648462311528E-14, 0.000000000000000000 ) ) ;
#11517=VERTEX_POINT ( 'NONE', #59488 ) ;
#11520=ORIENTED_EDGE ( 'NONE', *, *, #67129, .T. ) ;
#11547=VERTEX_POINT ( 'NONE', #11298 ) ;
#11558=VECTOR ( 'NONE', #11037, 1000.000000000000000 ) ;
#11569=CARTESIAN_POINT ( 'NONE',  ( 0.000000000000000000, 0.000000000000000000, 85.00000000000000000 ) ) ;
#11608=CIRCLE ( 'NONE', #68900, 74.99999999999998579 ) ;
#11612=CARTESIAN_POINT ( 'NONE',  ( 10.55634918610397577, -26.11269837220809364, 85.00100000000000477 ) ) ;
#11628=ORIENTED_EDGE ( 'NONE', *, *, #69087, .T. ) ;
#11633=DIRECTION ( 'NONE',  ( 0.000000000000000000, 0.000000000000000000, 1.000000000000000000 ) ) ;
#11685=CARTESIAN_POINT ( 'NONE',  ( 31.11269837220800127, -31.11269837220812562, 85.00100000000000477 ) ) ;
#11689=EDGE_CURVE ( 'NONE', #192, #7572, #65842, .T. ) ;
#11694=VECTOR ( 'NONE', #27800, 1000.000000000000000 ) ;
#11696=CARTESIAN_POINT ( 'NONE',  ( -5.000000000000058620, -31.11269837220806878, 2.000000000000001776 ) ) ;
#11705=VECTOR ( 'NONE', #14627, 1000.000000000000000 ) ;
#11712=LINE ( 'NONE', #50053, #58748 ) ;
#11722=CARTESIAN_POINT ( 'NONE',  ( 6.375108774214766072E-14, 31.11269837220806167, 85.00100000000000477 ) ) ;
#11731=CARTESIAN_POINT ( 'NONE',  ( -4.999999999999922728, 46.66904755831208718, 0.000000000000000000 ) ) ;
#11732=EDGE_LOOP ( 'NONE', ( #15192, #67050, #64033, #53010 ) ) ;
#11768=ORIENTED_EDGE ( 'NONE', *, *, #57745, .F. ) ;
#11781=DIRECTION ( 'NONE',  ( 1.000000000000000000, 0.000000000000000000, 0.000000000000000000 ) ) ;
#11798=LINE ( 'NONE', #6536, #64524 ) ;
#11830=ORIENTED_EDGE ( 'NONE', *, *, #19401, .T. ) ;
#11884=ORIENTED_EDGE ( 'NONE', *, *, #67906, .T. ) ;
#11900=ADVANCED_FACE ( 'NONE', ( #30624 ), #3535, .F. ) ;
#11967=VERTEX_POINT ( 'NONE', #63323 ) ;
#11977=ORIENTED_EDGE ( 'NONE', *, *, #32971, .F. ) ;
#11979=EDGE_CURVE ( 'NONE', #21301, #16538, #15131, .T. ) ;
#11992=EDGE_CURVE ( 'NONE', #53816, #62932, #6296, .T. ) ;
#12019=ADVANCED_FACE ( 'NONE', ( #32347 ), #53084, .F. ) ;
#12025=DIRECTION ( 'NONE',  ( 0.000000000000000000, 1.000000000000000000, -0.000000000000000000 ) ) ;
#12035=CARTESIAN_POINT ( 'NONE',  ( -20.55634918610411077, -41.66904755831209428, 2.000000000000001776 ) ) ;
#12040=ORIENTED_EDGE ( 'NONE', *, *, #2084, .T. ) ;
#12046=DIRECTION ( 'NONE',  ( -1.000000000000000000, 0.000000000000000000, 0.000000000000000000 ) ) ;
#12047=VECTOR ( 'NONE', #5888, 1000.000000000000000 ) ;
#12048=ORIENTED_EDGE ( 'NONE', *, *, #6511, .T. ) ;
#12054=EDGE_CURVE ( 'NONE', #44813, #11517, #5594, .T. ) ;
#12059=VERTEX_POINT ( 'NONE', #48832 ) ;
#12064=VECTOR ( 'NONE', #26160, 1000.000000000000000 ) ;
#12075=CARTESIAN_POINT ( 'NONE',  ( -36.11269837220806522, 5.594483210025202879E-14, 85.00100000000000477 ) ) ;
#12082=ADVANCED_FACE ( 'NONE', ( #56222 ), #51347, .T. ) ;
#12097=FILL_AREA_STYLE_COLOUR ( '', #43955 ) ;
#12105=LINE ( 'NONE', #18080, #19464 ) ;
#12115=AXIS2_PLACEMENT_3D ( 'NONE', #67006, #8601, #3312 ) ;
#12126=DIRECTION ( 'NONE',  ( 1.000000000000000000, 0.000000000000000000, 0.000000000000000000 ) ) ;
#12168=ORIENTED_EDGE ( 'NONE', *, *, #47153, .T. ) ;
#12179=ORIENTED_EDGE ( 'NONE', *, *, #50604, .F. ) ;
#12183=LINE ( 'NONE', #23085, #26681 ) ;
#12189=EDGE_CURVE ( 'NONE', #18870, #67789, #45680, .T. ) ;
#12190=FACE_OUTER_BOUND ( 'NONE', #62376, .T. ) ;
#12195=DIRECTION ( 'NONE',  ( 0.000000000000000000, -1.000000000000000000, 0.000000000000000000 ) ) ;
#12204=ORIENTED_EDGE ( 'NONE', *, *, #5483, .T. ) ;
#12211=AXIS2_PLACEMENT_3D ( 'NONE', #6861, #65977, #55386 ) ;
#12232=EDGE_CURVE ( 'NONE', #27095, #56869, #26641, .T. ) ;
#12242=EDGE_CURVE ( 'NONE', #58547, #40273, #69531, .T. ) ;
#12268=ORIENTED_EDGE ( 'NONE', *, *, #2084, .F. ) ;
#12273=CARTESIAN_POINT ( 'NONE',  ( -36.11269837220804391, 20.55634918610408945, 0.000000000000000000 ) ) ;
#12274=PLANE ( 'NONE',  #28789 ) ;
#12282=CARTESIAN_POINT ( 'NONE',  ( -31.11269837220806878, 5.000000000000056843, 2.000000000000001776 ) ) ;
#12317=ORIENTED_EDGE ( 'NONE', *, *, #47261, .F. ) ;
#12342=VECTOR ( 'NONE', #48912, 1000.000000000000000 ) ;
#12370=CARTESIAN_POINT ( 'NONE',  ( 31.11269837220806522, -6.375108774214766072E-14, 85.00100000000000477 ) ) ;
#12383=FACE_OUTER_BOUND ( 'NONE', #58298, .T. ) ;
#12393=CARTESIAN_POINT ( 'NONE',  ( -51.66904755831212981, -15.55634918610397222, 0.000000000000000000 ) ) ;
#12446=VECTOR ( 'NONE', #36680, 1000.000000000000000 ) ;
#12467=DIRECTION ( 'NONE',  ( -0.000000000000000000, -0.000000000000000000, -1.000000000000000000 ) ) ;
#12473=EDGE_CURVE ( 'NONE', #4596, #53834, #60856, .T. ) ;
#12482=VECTOR ( 'NONE', #4100, 1000.000000000000000 ) ;
#12488=VERTEX_POINT ( 'NONE', #55227 ) ;
#12496=VECTOR ( 'NONE', #52986, 1000.000000000000000 ) ;
#12497=EDGE_CURVE ( 'NONE', #39103, #46320, #17244, .T. ) ;
#12540=CARTESIAN_POINT ( 'NONE',  ( -31.11269837220809364, -15.55634918610397754, 0.000000000000000000 ) ) ;
#12545=STYLED_ITEM ( 'NONE', ( #54284 ), #16293 ) ;
#12581=AXIS2_PLACEMENT_3D ( 'NONE', #5902, #54435, #10846 ) ;
#12583=ORIENTED_EDGE ( 'NONE', *, *, #67031, .T. ) ;
#12597=FACE_BOUND ( 'NONE', #39765, .T. ) ;
#12600=CARTESIAN_POINT ( 'NONE',  ( 0.000000000000000000, 5.000000000000000000, 2.000000000000001776 ) ) ;
#12645=EDGE_CURVE ( 'NONE', #63246, #16366, #42603, .T. ) ;
#12647=ORIENTED_EDGE ( 'NONE', *, *, #2837, .F. ) ;
#12649=LINE ( 'NONE', #55545, #62635 ) ;
#12650=EDGE_LOOP ( 'NONE', ( #64800, #1066, #39049, #26063 ) ) ;
#12652=CARTESIAN_POINT ( 'NONE',  ( 26.11269837220809364, 15.55634918610396866, 0.000000000000000000 ) ) ;
#12675=CARTESIAN_POINT ( 'NONE',  ( 2.905661822261151883E-14, 20.55634918610402906, 0.000000000000000000 ) ) ;
#12698=CYLINDRICAL_SURFACE ( 'NONE', #41552, 66.50000000000000000 ) ;
#12706=DIRECTION ( 'NONE',  ( -0.000000000000000000, -0.000000000000000000, -1.000000000000000000 ) ) ;
#12709=DIRECTION ( 'NONE',  ( 0.000000000000000000, 1.000000000000000000, -0.000000000000000000 ) ) ;
#12726=EDGE_CURVE ( 'NONE', #11163, #11222, #1083, .T. ) ;
#12729=ORIENTED_EDGE ( 'NONE', *, *, #35915, .T. ) ;
#12775=ORIENTED_EDGE ( 'NONE', *, *, #29341, .T. ) ;
#12793=VECTOR ( 'NONE', #14214, 1000.000000000000000 ) ;
#12801=EDGE_CURVE ( 'NONE', #30210, #58410, #28151, .T. ) ;
#12813=EDGE_CURVE ( 'NONE', #51672, #64960, #59807, .T. ) ;
#12819=EDGE_CURVE ( 'NONE', #23331, #35061, #33095, .T. ) ;
#12825=LINE ( 'NONE', #53187, #68882 ) ;
#12867=ORIENTED_EDGE ( 'NONE', *, *, #35697, .F. ) ;
#12883=ADVANCED_FACE ( 'NONE', ( #44330 ), #65817, .F. ) ;
#12884=CARTESIAN_POINT ( 'NONE',  ( 10.55634918610397577, -31.11269837220809364, 2.000000000000000000 ) ) ;
#12900=LINE ( 'NONE', #34704, #47549 ) ;
#12921=CARTESIAN_POINT ( 'NONE',  ( 15.55634918610397399, -31.11269837220809364, 2.000000000000001776 ) ) ;
#12932=VERTEX_POINT ( 'NONE', #24983 ) ;
#12952=DIRECTION ( 'NONE',  ( -0.000000000000000000, -0.000000000000000000, -1.000000000000000000 ) ) ;
#12963=ORIENTED_EDGE ( 'NONE', *, *, #4208, .F. ) ;
#12976=AXIS2_PLACEMENT_3D ( 'NONE', #51362, #18657, #35529 ) ;
#12978=CARTESIAN_POINT ( 'NONE',  ( -20.55634918610411077, -46.66904755831208718, 85.00100000000000477 ) ) ;
#13014=CARTESIAN_POINT ( 'NONE',  ( 15.55634918610396511, -41.66904755831214402, 2.000000000000001776 ) ) ;
#13064=DIRECTION ( 'NONE',  ( -1.000000000000000000, 0.000000000000000000, 0.000000000000000000 ) ) ;
#13107=LINE ( 'NONE', #13446, #296 ) ;
#13132=VECTOR ( 'NONE', #36358, 1000.000000000000000 ) ;
#13144=ORIENTED_EDGE ( 'NONE', *, *, #66345, .T. ) ;
#13171=PLANE ( 'NONE',  #23970 ) ;
#13195=LINE ( 'NONE', #34659, #4378 ) ;
#13227=ORIENTED_EDGE ( 'NONE', *, *, #41695, .F. ) ;
#13244=LINE ( 'NONE', #28363, #49866 ) ;
#13267=ORIENTED_EDGE ( 'NONE', *, *, #41674, .T. ) ;
#13282=ADVANCED_FACE ( 'NONE', ( #38198 ), #43465, .F. ) ;
#13310=ORIENTED_EDGE ( 'NONE', *, *, #30054, .T. ) ;
#13315=DIRECTION ( 'NONE',  ( -0.000000000000000000, -0.000000000000000000, -1.000000000000000000 ) ) ;
#13332=EDGE_LOOP ( 'NONE', ( #25977, #62672, #12040, #27905 ) ) ;
#13349=ORIENTED_EDGE ( 'NONE', *, *, #67439, .T. ) ;
#13365=ORIENTED_EDGE ( 'NONE', *, *, #3014, .T. ) ;
#13368=ORIENTED_EDGE ( 'NONE', *, *, #150, .T. ) ;
#13372=VERTEX_POINT ( 'NONE', #30345 ) ;
#13387=VERTEX_POINT ( 'NONE', #2921 ) ;
#13393=CARTESIAN_POINT ( 'NONE',  ( -5.767955557622883589E-14, -31.11269837220806878, 0.000000000000000000 ) ) ;
#13424=AXIS2_PLACEMENT_3D ( 'NONE', #38160, #34296, #23402 ) ;
#13427=LINE ( 'NONE', #39127, #66473 ) ;
#13428=LINE ( 'NONE', #6753, #66714 ) ;
#13435=DIRECTION ( 'NONE',  ( 0.000000000000000000, 0.000000000000000000, -1.000000000000000000 ) ) ;
#13446=CARTESIAN_POINT ( 'NONE',  ( 31.11269837220800127, -31.11269837220812562, 2.000000000000001776 ) ) ;
#13459=EDGE_CURVE ( 'NONE', #2018, #65364, #46864, .T. ) ;
#13460=LINE ( 'NONE', #3255, #8773 ) ;
#13463=DIRECTION ( 'NONE',  ( 0.000000000000000000, -1.000000000000000000, 0.000000000000000000 ) ) ;
#13484=ORIENTED_EDGE ( 'NONE', *, *, #14702, .T. ) ;
#13497=EDGE_CURVE ( 'NONE', #39680, #59960, #48556, .T. ) ;
#13506=VECTOR ( 'NONE', #56837, 1000.000000000000000 ) ;
#13508=ORIENTED_EDGE ( 'NONE', *, *, #25356, .F. ) ;
#13523=CARTESIAN_POINT ( 'NONE',  ( -15.55634918610411077, -46.66904755831208718, 0.000000000000000000 ) ) ;
#13528=CARTESIAN_POINT ( 'NONE',  ( 6.375108774214766072E-14, 31.11269837220806167, 0.000000000000000000 ) ) ;
#13532=ORIENTED_EDGE ( 'NONE', *, *, #31587, .T. ) ;
#13533=VERTEX_POINT ( 'NONE', #21498 ) ;
#13548=CARTESIAN_POINT ( 'NONE',  ( 10.55634918610400419, -15.55634918610406103, 0.000000000000000000 ) ) ;
#13562=DIRECTION ( 'NONE',  ( 1.000000000000000000, -0.000000000000000000, 0.000000000000000000 ) ) ;
#13575=EDGE_CURVE ( 'NONE', #41022, #10664, #5662, .T. ) ;
#13581=DIRECTION ( 'NONE',  ( -0.000000000000000000, -1.000000000000000000, -0.000000000000000000 ) ) ;
#13608=DIRECTION ( 'NONE',  ( 0.000000000000000000, 0.000000000000000000, 1.000000000000000000 ) ) ;
#13613=CARTESIAN_POINT ( 'NONE',  ( 26.11269837220800127, -26.11269837220812562, 0.000000000000000000 ) ) ;
#13617=DIRECTION ( 'NONE',  ( 0.000000000000000000, 0.000000000000000000, 1.000000000000000000 ) ) ;
#13661=DIRECTION ( 'NONE',  ( 0.000000000000000000, 0.000000000000000000, -1.000000000000000000 ) ) ;
#13667=ORIENTED_EDGE ( 'NONE', *, *, #15498, .F. ) ;
#13695=LINE ( 'NONE', #51338, #5425 ) ;
#13713=VERTEX_POINT ( 'NONE', #10176 ) ;
#13743=CARTESIAN_POINT ( 'NONE',  ( 15.55634918610403261, 4.999999999999969802, 2.000000000000001776 ) ) ;
#13753=ORIENTED_EDGE ( 'NONE', *, *, #50004, .F. ) ;
#13758=DIRECTION ( 'NONE',  ( -0.000000000000000000, -0.000000000000000000, -1.000000000000000000 ) ) ;
#13772=CARTESIAN_POINT ( 'NONE',  ( -7.329206686002009974E-14, -41.66904755831212270, 2.000000000000001776 ) ) ;
#13782=VERTEX_POINT ( 'NONE', #6282 ) ;
#13787=CARTESIAN_POINT ( 'NONE',  ( 31.11269837220812562, 31.11269837220800483, 85.00100000000000477 ) ) ;
#13793=CARTESIAN_POINT ( 'NONE',  ( -15.55634918610408945, -31.11269837220804035, 85.00100000000000477 ) ) ;
#13814=PLANE ( 'NONE',  #39888 ) ;
#13825=AXIS2_PLACEMENT_3D ( 'NONE', #28893, #55259, #54196 ) ;
#13853=CARTESIAN_POINT ( 'NONE',  ( -15.55634918610403439, 2.818925648462311528E-14, 2.000000000000001776 ) ) ;
#13855=ORIENTED_EDGE ( 'NONE', *, *, #9200, .T. ) ;
#13859=CARTESIAN_POINT ( 'NONE',  ( -5.000000000000000000, 0.000000000000000000, 0.000000000000000000 ) ) ;
#13861=LINE ( 'NONE', #35323, #60317 ) ;
#13862=ORIENTED_EDGE ( 'NONE', *, *, #36875, .T. ) ;
#13879=VECTOR ( 'NONE', #44061, 1000.000000000000000 ) ;
#13883=VECTOR ( 'NONE', #45085, 999.9999999999998863 ) ;
#13890=CARTESIAN_POINT ( 'NONE',  ( -15.55634918610405748, -10.55634918610400597, 85.00100000000000477 ) ) ;
#13891=EDGE_LOOP ( 'NONE', ( #69246, #28459, #17873, #46797 ) ) ;
#13893=ORIENTED_EDGE ( 'NONE', *, *, #40169, .F. ) ;
#13906=EDGE_CURVE ( 'NONE', #31701, #59178, #51295, .T. ) ;
#13909=DIRECTION ( 'NONE',  ( -1.000000000000000000, 0.000000000000000000, 0.000000000000000000 ) ) ;
#13913=PLANE ( 'NONE',  #57 ) ;
#13938=CARTESIAN_POINT ( 'NONE',  ( -7.329206686002009974E-14, -46.66904755831211560, 0.000000000000000000 ) ) ;
#13940=VECTOR ( 'NONE', #19667, 1000.000000000000000 ) ;
#13941=ORIENTED_EDGE ( 'NONE', *, *, #5483, .F. ) ;
#13966=EDGE_CURVE ( 'NONE', #62805, #65715, #40039, .T. ) ;
#13980=ORIENTED_EDGE ( 'NONE', *, *, #51176, .F. ) ;
#13996=CARTESIAN_POINT ( 'NONE',  ( 26.11269837220803325, -10.55634918610409656, 0.000000000000000000 ) ) ;
#14017=LINE ( 'NONE', #67491, #47413 ) ;
#14030=ORIENTED_EDGE ( 'NONE', *, *, #49798, .F. ) ;
#14042=ORIENTED_EDGE ( 'NONE', *, *, #43838, .F. ) ;
#14051=ORIENTED_EDGE ( 'NONE', *, *, #61615, .T. ) ;
#14100=DIRECTION ( 'NONE',  ( -0.6246950475544236214, 7.650307904307285654E-17, 0.7808688094430308313 ) ) ;
#14102=VERTEX_POINT ( 'NONE', #37172 ) ;
#14107=CARTESIAN_POINT ( 'NONE',  ( 0.000000000000000000, 0.000000000000000000, 25.70156211871649887 ) ) ;
#14117=ADVANCED_FACE ( 'NONE', ( #33302 ), #38213, .F. ) ;
#14119=ORIENTED_EDGE ( 'NONE', *, *, #12232, .F. ) ;
#14124=DIRECTION ( 'NONE',  ( 0.000000000000000000, 0.000000000000000000, 1.000000000000000000 ) ) ;
#14133=VECTOR ( 'NONE', #118, 1000.000000000000000 ) ;
#14138=ORIENTED_EDGE ( 'NONE', *, *, #7943, .T. ) ;
#14163=DIRECTION ( 'NONE',  ( 0.000000000000000000, -0.000000000000000000, -1.000000000000000000 ) ) ;
#14203=DIRECTION ( 'NONE',  ( -1.000000000000000000, 0.000000000000000000, 0.000000000000000000 ) ) ;
#14214=DIRECTION ( 'NONE',  ( 0.000000000000000000, 1.000000000000000000, 0.000000000000000000 ) ) ;
#14219=EDGE_CURVE ( 'NONE', #24929, #53581, #28355, .T. ) ;
#14227=DIRECTION ( 'NONE',  ( 0.000000000000000000, 1.000000000000000000, 0.000000000000000000 ) ) ;
#14228=ORIENTED_EDGE ( 'NONE', *, *, #35915, .F. ) ;
#14249=ORIENTED_EDGE ( 'NONE', *, *, #22782, .T. ) ;
#14251=ORIENTED_EDGE ( 'NONE', *, *, #68387, .T. ) ;
#14252=DIRECTION ( 'NONE',  ( 0.000000000000000000, 0.000000000000000000, 1.000000000000000000 ) ) ;
#14260=CARTESIAN_POINT ( 'NONE',  ( 26.11269837220809364, 20.55634918610396866, 0.000000000000000000 ) ) ;
#14273=ORIENTED_EDGE ( 'NONE', *, *, #22782, .F. ) ;
#14282=VECTOR ( 'NONE', #44130, 1000.000000000000000 ) ;
#14308=ORIENTED_EDGE ( 'NONE', *, *, #40169, .T. ) ;
#14314=EDGE_CURVE ( 'NONE', #48274, #56852, #63145, .T. ) ;
#14323=ORIENTED_EDGE ( 'NONE', *, *, #33180, .F. ) ;
#14332=FACE_BOUND ( 'NONE', #37301, .T. ) ;
#14337=EDGE_CURVE ( 'NONE', #26154, #23331, #24490, .T. ) ;
#14346=CARTESIAN_POINT ( 'NONE',  ( 15.55634918610409656, 31.11269837220803325, 0.000000000000000000 ) ) ;
#14347=CARTESIAN_POINT ( 'NONE',  ( 46.66904755831207297, -10.55634918610412853, 85.00100000000000477 ) ) ;
#14348=DIRECTION ( 'NONE',  ( 1.000000000000000000, -0.000000000000000000, -0.000000000000000000 ) ) ;
#14369=VECTOR ( 'NONE', #37830, 1000.000000000000000 ) ;
#14383=AXIS2_PLACEMENT_3D ( 'NONE', #44916, #18536, #46292 ) ;
#14390=VECTOR ( 'NONE', #20986, 1000.000000000000000 ) ;
#14428=ORIENTED_EDGE ( 'NONE', *, *, #53094, .T. ) ;
#14452=ORIENTED_EDGE ( 'NONE', *, *, #25350, .F. ) ;
#14453=EDGE_LOOP ( 'NONE', ( #67858, #69247, #37240, #68009 ) ) ;
#14461=ORIENTED_EDGE ( 'NONE', *, *, #51380, .F. ) ;
#14529=ORIENTED_EDGE ( 'NONE', *, *, #13906, .F. ) ;
#14568=DIRECTION ( 'NONE',  ( 0.000000000000000000, -0.000000000000000000, -1.000000000000000000 ) ) ;
#14582=CARTESIAN_POINT ( 'NONE',  ( 15.55634918610396511, -46.66904755831214402, 85.00100000000000477 ) ) ;
#14607=EDGE_CURVE ( 'NONE', #5602, #7572, #49712, .T. ) ;
#14627=DIRECTION ( 'NONE',  ( 0.000000000000000000, 0.000000000000000000, 1.000000000000000000 ) ) ;
#14644=DIRECTION ( 'NONE',  ( 0.000000000000000000, 0.000000000000000000, 1.000000000000000000 ) ) ;
#14655=EDGE_LOOP ( 'NONE', ( #49700, #27053, #24923, #65784 ) ) ;
#14659=ORIENTED_EDGE ( 'NONE', *, *, #68405, .T. ) ;
#14674=ORIENTED_EDGE ( 'NONE', *, *, #61464, .T. ) ;
#14691=LINE ( 'NONE', #41086, #41990 ) ;
#14702=EDGE_CURVE ( 'NONE', #46372, #35681, #34952, .T. ) ;
#14714=VERTEX_POINT ( 'NONE', #29666 ) ;
#14745=CARTESIAN_POINT ( 'NONE',  ( 46.66904755831212981, 15.55634918610394379, 85.00100000000000477 ) ) ;
#14764=CARTESIAN_POINT ( 'NONE',  ( -4.999999999999936939, 31.11269837220806167, 85.00100000000000477 ) ) ;
#14778=LINE ( 'NONE', #25358, #171 ) ;
#14795=VERTEX_POINT ( 'NONE', #6298 ) ;
#14825=EDGE_CURVE ( 'NONE', #13533, #26941, #38304, .T. ) ;
#14826=VECTOR ( 'NONE', #47529, 1000.000000000000000 ) ;
#14830=EDGE_CURVE ( 'NONE', #10200, #16148, #22129, .T. ) ;
#14854=ORIENTED_EDGE ( 'NONE', *, *, #33936, .F. ) ;
#14859=DIRECTION ( 'NONE',  ( -1.000000000000000000, 0.000000000000000000, 0.000000000000000000 ) ) ;
#14864=CARTESIAN_POINT ( 'NONE',  ( 46.66904755831210139, -9.150666335777657423E-14, 0.000000000000000000 ) ) ;
#14874=CARTESIAN_POINT ( 'NONE',  ( 26.11269837220800127, -31.11269837220812562, 85.00100000000000477 ) ) ;
#14884=VECTOR ( 'NONE', #9438, 1000.000000000000000 ) ;
#14893=PLANE ( 'NONE',  #15375 ) ;
#14903=EDGE_LOOP ( 'NONE', ( #20656, #40521, #54008, #48187 ) ) ;
#14913=CARTESIAN_POINT ( 'NONE',  ( -15.55634918610408945, -31.11269837220804035, 0.000000000000000000 ) ) ;
#14992=CARTESIAN_POINT ( 'NONE',  ( 10.55634918610396511, -41.66904755831214402, 85.00100000000000477 ) ) ;
#15011=LINE ( 'NONE', #31883, #31948 ) ;
#15012=DIRECTION ( 'NONE',  ( 0.000000000000000000, 0.000000000000000000, 1.000000000000000000 ) ) ;
#15023=VECTOR ( 'NONE', #12195, 1000.000000000000000 ) ;
#15028=EDGE_CURVE ( 'NONE', #41430, #67865, #57622, .T. ) ;
#15040=VECTOR ( 'NONE', #4679, 1000.000000000000000 ) ;
#15044=VECTOR ( 'NONE', #57995, 1000.000000000000000 ) ;
#15062=LINE ( 'NONE', #36173, #16470 ) ;
#15089=LINE ( 'NONE', #5217, #60939 ) ;
#15108=CARTESIAN_POINT ( 'NONE',  ( 31.11269837220803325, -15.55634918610409656, 0.000000000000000000 ) ) ;
#15131=LINE ( 'NONE', #25006, #64837 ) ;
#15151=ORIENTED_EDGE ( 'NONE', *, *, #30050, .T. ) ;
#15157=EDGE_CURVE ( 'NONE', #33686, #37117, #10449, .T. ) ;
#15159=ORIENTED_EDGE ( 'NONE', *, *, #31755, .T. ) ;
#15169=VERTEX_POINT ( 'NONE', #43146 ) ;
#15192=ORIENTED_EDGE ( 'NONE', *, *, #46964, .T. ) ;
#15206=ORIENTED_EDGE ( 'NONE', *, *, #28604, .T. ) ;
#15209=FACE_OUTER_BOUND ( 'NONE', #56149, .T. ) ;
#15217=LINE ( 'NONE', #52505, #21746 ) ;
#15229=VECTOR ( 'NONE', #49456, 1000.000000000000000 ) ;
#15239=AXIS2_PLACEMENT_3D ( 'NONE', #14582, #3003, #30769 ) ;
#15242=EDGE_CURVE ( 'NONE', #67479, #11433, #59666, .T. ) ;
#15247=EDGE_CURVE ( 'NONE', #23032, #53816, #42801, .T. ) ;
#15278=ORIENTED_EDGE ( 'NONE', *, *, #12813, .F. ) ;
#15305=ORIENTED_EDGE ( 'NONE', *, *, #37282, .F. ) ;
#15310=CARTESIAN_POINT ( 'NONE',  ( -15.55634918610405748, -15.55634918610400774, 85.00100000000000477 ) ) ;
#15333=CARTESIAN_POINT ( 'NONE',  ( -36.11269837220809364, -15.55634918610397754, 0.000000000000000000 ) ) ;
#15337=ORIENTED_EDGE ( 'NONE', *, *, #54278, .T. ) ;
#15375=AXIS2_PLACEMENT_3D ( 'NONE', #46911, #40592, #41295 ) ;
#15404=EDGE_CURVE ( 'NONE', #51157, #64323, #56487, .T. ) ;
#15407=LINE ( 'NONE', #58306, #4086 ) ;
#15438=ORIENTED_EDGE ( 'NONE', *, *, #26708, .T. ) ;
#15439=VECTOR ( 'NONE', #64755, 1000.000000000000000 ) ;
#15441=ORIENTED_EDGE ( 'NONE', *, *, #11098, .T. ) ;
#15444=CARTESIAN_POINT ( 'NONE',  ( -15.55634918610411077, -46.66904755831208718, 85.00100000000000477 ) ) ;
#15459=ORIENTED_EDGE ( 'NONE', *, *, #1674, .T. ) ;
#15461=VERTEX_POINT ( 'NONE', #64882 ) ;
#15480=DIRECTION ( 'NONE',  ( 1.000000000000000000, -0.000000000000000000, -0.000000000000000000 ) ) ;
#15487=ORIENTED_EDGE ( 'NONE', *, *, #23985, .T. ) ;
#15493=CARTESIAN_POINT ( 'NONE',  ( 2.905661822261151883E-14, 20.55634918610402906, 0.000000000000000000 ) ) ;
#15498=EDGE_CURVE ( 'NONE', #21309, #25475, #15654, .T. ) ;
#15510=CARTESIAN_POINT ( 'NONE',  ( -15.55634918610405748, -15.55634918610400774, 85.00100000000000477 ) ) ;
#15579=DIRECTION ( 'NONE',  ( -0.000000000000000000, -0.000000000000000000, -1.000000000000000000 ) ) ;
#15629=CARTESIAN_POINT ( 'NONE',  ( -31.11269837220812207, -26.11269837220801193, 85.00100000000000477 ) ) ;
#15647=ORIENTED_EDGE ( 'NONE', *, *, #25925, .T. ) ;
#15654=LINE ( 'NONE', #64528, #19166 ) ;
#15675=VECTOR ( 'NONE', #41384, 1000.000000000000000 ) ;
#15700=ORIENTED_EDGE ( 'NONE', *, *, #53146, .T. ) ;
#15716=CARTESIAN_POINT ( 'NONE',  ( 0.000000000000000000, 0.000000000000000000, -0.002000000000002000178 ) ) ;
#15718=CARTESIAN_POINT ( 'NONE',  ( -31.11269837220804035, 15.55634918610408945, 85.00100000000000477 ) ) ;
#15744=CARTESIAN_POINT ( 'NONE',  ( 31.11269837220806522, -6.375108774214766072E-14, 85.00100000000000477 ) ) ;
#15748=CARTESIAN_POINT ( 'NONE',  ( 10.55634918610406281, 20.55634918610400064, 0.000000000000000000 ) ) ;
#15772=EDGE_CURVE ( 'NONE', #1617, #58260, #62349, .T. ) ;
#15780=ORIENTED_EDGE ( 'NONE', *, *, #4611, .F. ) ;
#15785=VERTEX_POINT ( 'NONE', #42272 ) ;
#15794=DIRECTION ( 'NONE',  ( 0.000000000000000000, 0.000000000000000000, -1.000000000000000000 ) ) ;
#15804=CARTESIAN_POINT ( 'NONE',  ( 41.66904755831210849, 4.999999999999909406, 85.00100000000000477 ) ) ;
#15822=DIRECTION ( 'NONE',  ( 0.000000000000000000, 1.000000000000000000, -0.000000000000000000 ) ) ;
#15829=CARTESIAN_POINT ( 'NONE',  ( -36.11269837220812207, -26.11269837220801193, 2.000000000000001776 ) ) ;
#15840=VECTOR ( 'NONE', #44939, 1000.000000000000000 ) ;
#15842=EDGE_LOOP ( 'NONE', ( #39117, #14051, #28964, #9589 ) ) ;
#15845=DIRECTION ( 'NONE',  ( -0.000000000000000000, -0.000000000000000000, -1.000000000000000000 ) ) ;
#15858=ORIENTED_EDGE ( 'NONE', *, *, #5245, .T. ) ;
#15874=VECTOR ( 'NONE', #39729, 1000.000000000000000 ) ;
#15890=VERTEX_POINT ( 'NONE', #38028 ) ;
#15893=CARTESIAN_POINT ( 'NONE',  ( 31.11269837220809364, 15.55634918610396866, 2.000000000000001776 ) ) ;
#15938=VECTOR ( 'NONE', #6661, 1000.000000000000000 ) ;
#15941=CARTESIAN_POINT ( 'NONE',  ( 41.66904755831208007, -15.55634918610412853, 0.000000000000000000 ) ) ;
#15961=LINE ( 'NONE', #58861, #14133 ) ;
#15968=DIRECTION ( 'NONE',  ( -1.000000000000000000, 0.000000000000000000, 0.000000000000000000 ) ) ;
#15976=VECTOR ( 'NONE', #33431, 1000.000000000000000 ) ;
#15982=EDGE_CURVE ( 'NONE', #25475, #33134, #46686, .T. ) ;
#16006=CARTESIAN_POINT ( 'NONE',  ( 26.11269837220800127, -26.11269837220812207, 2.000000000000001776 ) ) ;
#16012=EDGE_CURVE ( 'NONE', #13713, #29482, #63903, .T. ) ;
#16018=ADVANCED_FACE ( 'NONE', ( #26618 ), #5159, .F. ) ;
#16027=CARTESIAN_POINT ( 'NONE',  ( 31.11269837220812562, 31.11269837220800483, 0.000000000000000000 ) ) ;
#16035=FACE_BOUND ( 'NONE', #33527, .T. ) ;
#16050=FACE_OUTER_BOUND ( 'NONE', #34830, .T. ) ;
#16051=DIRECTION ( 'NONE',  ( 0.000000000000000000, -0.000000000000000000, -1.000000000000000000 ) ) ;
#16067=ORIENTED_EDGE ( 'NONE', *, *, #54602, .T. ) ;
#16107=LINE ( 'NONE', #58321, #12047 ) ;
#16111=LINE ( 'NONE', #25992, #66781 ) ;
#16114=EDGE_LOOP ( 'NONE', ( #38458, #65320, #44956, #19694 ) ) ;
#16120=VECTOR ( 'NONE', #33391, 1000.000000000000000 ) ;
#16125=PLANE ( 'NONE',  #12581 ) ;
#16135=ORIENTED_EDGE ( 'NONE', *, *, #47340, .T. ) ;
#16136=ORIENTED_EDGE ( 'NONE', *, *, #59389, .T. ) ;
#16145=DIRECTION ( 'NONE',  ( 0.000000000000000000, 0.000000000000000000, -1.000000000000000000 ) ) ;
#16146=VERTEX_POINT ( 'NONE', #12884 ) ;
#16148=VERTEX_POINT ( 'NONE', #17083 ) ;
#16152=CARTESIAN_POINT ( 'NONE',  ( -15.55634918610396866, 36.11269837220808654, 2.000000000000001776 ) ) ;
#16160=FACE_OUTER_BOUND ( 'NONE', #18619, .T. ) ;
#16162=VERTEX_POINT ( 'NONE', #62093 ) ;
#16170=VECTOR ( 'NONE', #23098, 1000.000000000000000 ) ;
#16187=CARTESIAN_POINT ( 'NONE',  ( 7.762887554996211747E-14, 46.66904755831208718, 0.000000000000000000 ) ) ;
#16192=EDGE_CURVE ( 'NONE', #30657, #55128, #34690, .T. ) ;
#16212=DIRECTION ( 'NONE',  ( -1.000000000000000000, 0.000000000000000000, 0.000000000000000000 ) ) ;
#16213=CARTESIAN_POINT ( 'NONE',  ( -46.66904755831212981, -15.55634918610397222, 0.000000000000000000 ) ) ;
#16214=LINE ( 'NONE', #21485, #34986 ) ;
#16236=FACE_OUTER_BOUND ( 'NONE', #35562, .T. ) ;
#16254=DIRECTION ( 'NONE',  ( 0.000000000000000000, -1.000000000000000000, 0.000000000000000000 ) ) ;
#16271=VECTOR ( 'NONE', #58432, 1000.000000000000000 ) ;
#16273=CARTESIAN_POINT ( 'NONE',  ( -15.55634918610408945, -31.11269837220804035, 85.00100000000000477 ) ) ;
#16277=AXIS2_PLACEMENT_3D ( 'NONE', #62356, #30348, #19093 ) ;
#16287=CARTESIAN_POINT ( 'NONE',  ( 15.55634918610406103, 15.55634918610400241, 2.000000000000001776 ) ) ;
#16293=MANIFOLD_SOLID_BREP ( 'Extrude-Thin1', #64247 ) ;
#16308=ORIENTED_EDGE ( 'NONE', *, *, #13966, .T. ) ;
#16311=CARTESIAN_POINT ( 'NONE',  ( -5.000000000000000000, 0.000000000000000000, 85.00100000000000477 ) ) ;
#16317=ORIENTED_EDGE ( 'NONE', *, *, #54699, .T. ) ;
#16332=ORIENTED_EDGE ( 'NONE', *, *, #19845, .T. ) ;
#16333=AXIS2_PLACEMENT_3D ( 'NONE', #11362, #65909, #22276 ) ;
#16341=ORIENTED_EDGE ( 'NONE', *, *, #38765, .T. ) ;
#16349=EDGE_CURVE ( 'NONE', #27957, #3914, #64515, .T. ) ;
#16354=CARTESIAN_POINT ( 'NONE',  ( 74.99999999999998579, 9.184850993605147156E-15, 25.00000000000007816 ) ) ;
#16366=VERTEX_POINT ( 'NONE', #40219 ) ;
#16386=FACE_OUTER_BOUND ( 'NONE', #25743, .T. ) ;
#16394=ORIENTED_EDGE ( 'NONE', *, *, #45188, .F. ) ;
#16408=PRODUCT_DEFINITION ( 'UNKNOWN', '', #43332, #26815 ) ;
#16420=ADVANCED_FACE ( 'NONE', ( #50765 ), #66968, .F. ) ;
#16428=AXIS2_PLACEMENT_3D ( 'NONE', #41115, #4855, #68200 ) ;
#16429=VECTOR ( 'NONE', #63796, 1000.000000000000000 ) ;
#16431=DIRECTION ( 'NONE',  ( 1.000000000000000000, -0.000000000000000000, -0.000000000000000000 ) ) ;
#16433=VERTEX_POINT ( 'NONE', #41942 ) ;
#16436=PLANE ( 'NONE',  #4823 ) ;
#16440=VECTOR ( 'NONE', #36662, 1000.000000000000000 ) ;
#16452=ORIENTED_EDGE ( 'NONE', *, *, #20088, .T. ) ;
#16454=CARTESIAN_POINT ( 'NONE',  ( -15.55634918610411077, -46.66904755831208718, 0.000000000000000000 ) ) ;
#16470=VECTOR ( 'NONE', #5196, 1000.000000000000000 ) ;
#16489=CARTESIAN_POINT ( 'NONE',  ( 7.762887554996211747E-14, 51.66904755831208718, 0.000000000000000000 ) ) ;
#16506=DIRECTION ( 'NONE',  ( 0.000000000000000000, 0.000000000000000000, -1.000000000000000000 ) ) ;
#16507=CARTESIAN_POINT ( 'NONE',  ( -46.66904755831212981, -10.55634918610397222, 85.00100000000000477 ) ) ;
#16520=EDGE_CURVE ( 'NONE', #29447, #327, #3970, .T. ) ;
#16538=VERTEX_POINT ( 'NONE', #59140 ) ;
#16544=ORIENTED_EDGE ( 'NONE', *, *, #26581, .T. ) ;
#16549=ORIENTED_EDGE ( 'NONE', *, *, #55046, .T. ) ;
#16562=LINE ( 'NONE', #64058, #31608 ) ;
#16563=FACE_OUTER_BOUND ( 'NONE', #32019, .T. ) ;
#16569=CARTESIAN_POINT ( 'NONE',  ( 31.11269837220812562, 31.11269837220800483, 2.000000000000001776 ) ) ;
#16589=FACE_OUTER_BOUND ( 'NONE', #56342, .T. ) ;
#16642=CARTESIAN_POINT ( 'NONE',  ( -4.999999999999971578, 20.55634918610402906, 2.000000000000001776 ) ) ;
#16647=EDGE_LOOP ( 'NONE', ( #32546, #36119, #68266, #28589 ) ) ;
#16655=EDGE_CURVE ( 'NONE', #16958, #38815, #24660, .T. ) ;
#16664=EDGE_LOOP ( 'NONE', ( #35732, #42595, #2716, #42915 ) ) ;
#16669=EDGE_CURVE ( 'NONE', #69309, #32392, #34177, .T. ) ;
#16680=ADVANCED_FACE ( 'NONE', ( #62636 ), #47464, .F. ) ;
#16682=EDGE_CURVE ( 'NONE', #55179, #65524, #14778, .T. ) ;
#16693=LINE ( 'NONE', #37449, #33263 ) ;
#16716=FACE_OUTER_BOUND ( 'NONE', #17583, .T. ) ;
#16720=PLANE ( 'NONE',  #44599 ) ;
#16722=FACE_BOUND ( 'NONE', #46600, .T. ) ;
#16735=ADVANCED_FACE ( 'NONE', ( #57011 ), #35898, .F. ) ;
#16770=CARTESIAN_POINT ( 'NONE',  ( 31.11269837220806522, -6.375108774214766072E-14, 0.000000000000000000 ) ) ;
#16781=CARTESIAN_POINT ( 'NONE',  ( -36.11269837220809364, -15.55634918610397754, 2.000000000000001776 ) ) ;
#16788=CARTESIAN_POINT ( 'NONE',  ( 15.55634918610403261, -3.079134169858832593E-14, 2.000000000000001776 ) ) ;
#16819=EDGE_LOOP ( 'NONE', ( #21639, #37982, #55218, #3453 ) ) ;
#16821=ORIENTED_EDGE ( 'NONE', *, *, #42918, .F. ) ;
#16824=DIRECTION ( 'NONE',  ( 0.000000000000000000, -1.000000000000000000, 0.000000000000000000 ) ) ;
#16835=ORIENTED_EDGE ( 'NONE', *, *, #37296, .T. ) ;
#16847=ORIENTED_EDGE ( 'NONE', *, *, #54150, .F. ) ;
#16848=CARTESIAN_POINT ( 'NONE',  ( -15.55634918610408945, -31.11269837220804035, 85.00100000000000477 ) ) ;
#16850=ORIENTED_EDGE ( 'NONE', *, *, #25356, .T. ) ;
#16859=ORIENTED_EDGE ( 'NONE', *, *, #33602, .T. ) ;
#16863=PLANE ( 'NONE',  #64930 ) ;
#16894=CARTESIAN_POINT ( 'NONE',  ( 15.55634918610406103, 15.55634918610400241, 2.000000000000001776 ) ) ;
#16901=DIRECTION ( 'NONE',  ( -0.000000000000000000, -0.000000000000000000, -1.000000000000000000 ) ) ;
#16911=PLANE ( 'NONE',  #6591 ) ;
#16952=DIRECTION ( 'NONE',  ( 0.000000000000000000, 1.000000000000000000, -0.000000000000000000 ) ) ;
#16955=CARTESIAN_POINT ( 'NONE',  ( -15.55634918610396866, 31.11269837220809009, 2.000000000000001776 ) ) ;
#16958=VERTEX_POINT ( 'NONE', #18596 ) ;
#16989=MECHANICAL_DESIGN_GEOMETRIC_PRESENTATION_REPRESENTATION('',(#12545),#31618);
#16990=ORIENTED_EDGE ( 'NONE', *, *, #25293, .F. ) ;
#17004=SURFACE_SIDE_STYLE ('',( #1190 ) ) ;
#17041=ORIENTED_EDGE ( 'NONE', *, *, #39582, .T. ) ;
#17083=CARTESIAN_POINT ( 'NONE',  ( 15.55634918610400241, -10.55634918610406281, 2.000000000000001776 ) ) ;
#17101=CARTESIAN_POINT ( 'NONE',  ( 31.11269837220809364, 20.55634918610396866, 2.000000000000001776 ) ) ;
#17138=DIRECTION ( 'NONE',  ( 0.6246950475544236214, 0.000000000000000000, 0.7808688094430308313 ) ) ;
#17142=ORIENTED_EDGE ( 'NONE', *, *, #29637, .F. ) ;
#17215=VECTOR ( 'NONE', #2187, 1000.000000000000000 ) ;
#17229=FACE_OUTER_BOUND ( 'NONE', #68189, .T. ) ;
#17236=AXIS2_PLACEMENT_3D ( 'NONE', #42553, #15822, #37264 ) ;
#17244=LINE ( 'NONE', #49952, #47995 ) ;
#17255=VERTEX_POINT ( 'NONE', #7178 ) ;
#17260=LINE ( 'NONE', #14346, #59255 ) ;
#17285=ORIENTED_EDGE ( 'NONE', *, *, #22337, .T. ) ;
#17296=CARTESIAN_POINT ( 'NONE',  ( -31.11269837220806878, 5.594483210025202879E-14, 0.000000000000000000 ) ) ;
#17333=AXIS2_PLACEMENT_3D ( 'NONE', #16848, #21436, #32007 ) ;
#17363=CARTESIAN_POINT ( 'NONE',  ( -72.99999999999998579, 0.000000000000000000, 85.00000000000000000 ) ) ;
#17428=DIRECTION ( 'NONE',  ( -1.000000000000000000, 0.000000000000000000, 0.000000000000000000 ) ) ;
#17450=ORIENTED_EDGE ( 'NONE', *, *, #42234, .F. ) ;
#17462=DIRECTION ( 'NONE',  ( -1.000000000000000000, 0.000000000000000000, 0.000000000000000000 ) ) ;
#17472=ADVANCED_FACE ( 'NONE', ( #3626 ), #2258, .F. ) ;
#17474=VECTOR ( 'NONE', #59486, 1000.000000000000000 ) ;
#17478=ADVANCED_FACE ( 'NONE', ( #57104 ), #24057, .F. ) ;
#17484=CARTESIAN_POINT ( 'NONE',  ( -31.11269837220806878, 0.000000000000000000, 0.000000000000000000 ) ) ;
#17502=ORIENTED_EDGE ( 'NONE', *, *, #42918, .T. ) ;
#17503=DIRECTION ( 'NONE',  ( -0.000000000000000000, -0.000000000000000000, -1.000000000000000000 ) ) ;
#17504=CARTESIAN_POINT ( 'NONE',  ( -7.329206686002009974E-14, -41.66904755831212270, 2.000000000000001776 ) ) ;
#17510=VERTEX_POINT ( 'NONE', #62378 ) ;
#17514=VECTOR ( 'NONE', #46505, 1000.000000000000000 ) ;
#17516=DIRECTION ( 'NONE',  ( -0.000000000000000000, -0.000000000000000000, 1.000000000000000000 ) ) ;
#17537=ORIENTED_EDGE ( 'NONE', *, *, #37954, .T. ) ;
#17540=ORIENTED_EDGE ( 'NONE', *, *, #37282, .T. ) ;
#17555=CARTESIAN_POINT ( 'NONE',  ( -36.11269837220809364, -10.55634918610397932, 85.00100000000000477 ) ) ;
#17570=EDGE_CURVE ( 'NONE', #1454, #6738, #64794, .T. ) ;
#17575=CARTESIAN_POINT ( 'NONE',  ( -15.55634918610403439, 5.000000000000028422, 2.000000000000001776 ) ) ;
#17580=VECTOR ( 'NONE', #931, 1000.000000000000000 ) ;
#17581=ORIENTED_EDGE ( 'NONE', *, *, #54690, .T. ) ;
#17583=EDGE_LOOP ( 'NONE', ( #20389, #66667, #24078, #48547 ) ) ;
#17586=DIRECTION ( 'NONE',  ( 1.000000000000000000, 0.000000000000000000, -0.000000000000000000 ) ) ;
#17588=CARTESIAN_POINT ( 'NONE',  ( 26.11269837220806167, -6.375108774214766072E-14, 0.000000000000000000 ) ) ;
#17590=DIRECTION ( 'NONE',  ( 0.000000000000000000, -1.000000000000000000, 0.000000000000000000 ) ) ;
#17615=FACE_OUTER_BOUND ( 'NONE', #45884, .T. ) ;
#17621=DIRECTION ( 'NONE',  ( 0.000000000000000000, 0.000000000000000000, 1.000000000000000000 ) ) ;
#17639=VECTOR ( 'NONE', #43849, 1000.000000000000000 ) ;
#17650=CARTESIAN_POINT ( 'NONE',  ( -5.000000000000058620, -31.11269837220806878, 0.000000000000000000 ) ) ;
#17664=DIRECTION ( 'NONE',  ( -0.000000000000000000, -0.000000000000000000, 1.000000000000000000 ) ) ;
#17684=ORIENTED_EDGE ( 'NONE', *, *, #16682, .T. ) ;
#17712=CARTESIAN_POINT ( 'NONE',  ( -74.99999999999998579, 0.000000000000000000, 85.00000000000000000 ) ) ;
#17742=CARTESIAN_POINT ( 'NONE',  ( 2.905661822261151883E-14, 15.55634918610403084, 2.000000000000001776 ) ) ;
#17763=LINE ( 'NONE', #39217, #59096 ) ;
#17800=CARTESIAN_POINT ( 'NONE',  ( -72.99999999999998579, 0.000000000000000000, 25.70156211871649887 ) ) ;
#17807=EDGE_CURVE ( 'NONE', #62528, #42408, #59759, .T. ) ;
#17811=CARTESIAN_POINT ( 'NONE',  ( 54.99999999999995026, 0.000000000000000000, 0.000000000000000000 ) ) ;
#17818=VERTEX_POINT ( 'NONE', #42889 ) ;
#17852=VERTEX_POINT ( 'NONE', #44283 ) ;
#17865=DIRECTION ( 'NONE',  ( 1.000000000000000000, -0.000000000000000000, 0.000000000000000000 ) ) ;
#17867=ORIENTED_EDGE ( 'NONE', *, *, #36948, .F. ) ;
#17872=FACE_BOUND ( 'NONE', #20153, .T. ) ;
#17873=ORIENTED_EDGE ( 'NONE', *, *, #9597, .F. ) ;
#17881=AXIS2_PLACEMENT_3D ( 'NONE', #58938, #5817, #27628 ) ;
#17896=VERTEX_POINT ( 'NONE', #15748 ) ;
#17913=DIRECTION ( 'NONE',  ( 1.000000000000000000, 0.000000000000000000, 0.000000000000000000 ) ) ;
#17931=LINE ( 'NONE', #44999, #62993 ) ;
#17932=EDGE_LOOP ( 'NONE', ( #34840, #54443, #53824, #57914 ) ) ;
#17934=AXIS2_PLACEMENT_3D ( 'NONE', #21570, #37400, #5403 ) ;
#17951=ORIENTED_EDGE ( 'NONE', *, *, #47687, .F. ) ;
#17961=CARTESIAN_POINT ( 'NONE',  ( 26.11269837220800127, -31.11269837220812562, 0.000000000000000000 ) ) ;
#17964=DIRECTION ( 'NONE',  ( 0.000000000000000000, 0.000000000000000000, -1.000000000000000000 ) ) ;
#17989=CARTESIAN_POINT ( 'NONE',  ( -46.66904755831210139, 0.000000000000000000, 0.000000000000000000 ) ) ;
#17994=CARTESIAN_POINT ( 'NONE',  ( -31.11269837220812207, -31.11269837220801193, 0.000000000000000000 ) ) ;
#18011=LINE ( 'NONE', #39461, #51141 ) ;
#18025=ADVANCED_FACE ( 'NONE', ( #48861 ), #48173, .F. ) ;
#18032=DIRECTION ( 'NONE',  ( 0.000000000000000000, -1.000000000000000000, 0.000000000000000000 ) ) ;
#18069=VERTEX_POINT ( 'NONE', #48514 ) ;
#18078=DIRECTION ( 'NONE',  ( 0.000000000000000000, -1.000000000000000000, 0.000000000000000000 ) ) ;
#18080=CARTESIAN_POINT ( 'NONE',  ( -20.55634918610405748, -15.55634918610400774, 2.000000000000001776 ) ) ;
#18082=EDGE_LOOP ( 'NONE', ( #39911, #22805, #5836, #12268 ) ) ;
#18083=ORIENTED_EDGE ( 'NONE', *, *, #63136, .F. ) ;
#18102=CARTESIAN_POINT ( 'NONE',  ( 15.55634918610397399, -31.11269837220809364, 2.000000000000001776 ) ) ;
#18118=EDGE_CURVE ( 'NONE', #36200, #1187, #17931, .T. ) ;
#18123=CARTESIAN_POINT ( 'NONE',  ( -5.000000000000073719, -46.66904755831211560, 2.000000000000000000 ) ) ;
#18130=ORIENTED_EDGE ( 'NONE', *, *, #69308, .T. ) ;
#18136=ORIENTED_EDGE ( 'NONE', *, *, #41695, .T. ) ;
#18138=VERTEX_POINT ( 'NONE', #22505 ) ;
#18145=LINE ( 'NONE', #66696, #21894 ) ;
#18160=CARTESIAN_POINT ( 'NONE',  ( 15.55634918610397399, -31.11269837220809364, 85.00100000000000477 ) ) ;
#18164=ORIENTED_EDGE ( 'NONE', *, *, #23112, .F. ) ;
#18197=EDGE_CURVE ( 'NONE', #4486, #19070, #56251, .T. ) ;
#18222=ORIENTED_EDGE ( 'NONE', *, *, #39057, .F. ) ;
#18230=EDGE_LOOP ( 'NONE', ( #63511, #47058, #41676, #63 ) ) ;
#18233=DIRECTION ( 'NONE',  ( 1.000000000000000000, 0.000000000000000000, 0.000000000000000000 ) ) ;
#18238=CARTESIAN_POINT ( 'NONE',  ( 26.11269837220806167, 4.999999999999936939, 2.000000000000001776 ) ) ;
#18248=ADVANCED_FACE ( 'NONE', ( #49569 ), #1398, .F. ) ;
#18263=VECTOR ( 'NONE', #68671, 1000.000000000000000 ) ;
#18282=LINE ( 'NONE', #2803, #15976 ) ;
#18312=VECTOR ( 'NONE', #48647, 1000.000000000000000 ) ;
#18343=VECTOR ( 'NONE', #12709, 1000.000000000000000 ) ;
#18345=LINE ( 'NONE', #17296, #49879 ) ;
#18355=VECTOR ( 'NONE', #68024, 1000.000000000000000 ) ;
#18360=VECTOR ( 'NONE', #40304, 1000.000000000000000 ) ;
#18367=ORIENTED_EDGE ( 'NONE', *, *, #15242, .F. ) ;
#18377=ORIENTED_EDGE ( 'NONE', *, *, #1674, .F. ) ;
#18386=CARTESIAN_POINT ( 'NONE',  ( 31.11269837220803325, -10.55634918610409656, 85.00100000000000477 ) ) ;
#18422=ORIENTED_EDGE ( 'NONE', *, *, #67439, .F. ) ;
#18432=DIRECTION ( 'NONE',  ( -0.000000000000000000, -1.000000000000000000, -0.000000000000000000 ) ) ;
#18446=EDGE_LOOP ( 'NONE', ( #24342, #16850, #5267, #18222 ) ) ;
#18460=VECTOR ( 'NONE', #1582, 1000.000000000000000 ) ;
#18462=EDGE_LOOP ( 'NONE', ( #1534, #61505, #63091, #67080 ) ) ;
#18467=ORIENTED_EDGE ( 'NONE', *, *, #61492, .T. ) ;
#18531=VERTEX_POINT ( 'NONE', #57560 ) ;
#18536=DIRECTION ( 'NONE',  ( 0.000000000000000000, 1.000000000000000000, -0.000000000000000000 ) ) ;
#18541=CARTESIAN_POINT ( 'NONE',  ( -46.66904755831212981, -15.55634918610397222, 85.00100000000000477 ) ) ;
#18555=ORIENTED_EDGE ( 'NONE', *, *, #1826, .F. ) ;
#18556=ORIENTED_EDGE ( 'NONE', *, *, #26148, .F. ) ;
#18564=FACE_BOUND ( 'NONE', #33083, .T. ) ;
#18569=ADVANCED_FACE ( 'NONE', ( #29438 ), #9370, .F. ) ;
#18574=ORIENTED_EDGE ( 'NONE', *, *, #36060, .F. ) ;
#18575=ORIENTED_EDGE ( 'NONE', *, *, #46533, .F. ) ;
#18577=CARTESIAN_POINT ( 'NONE',  ( 0.000000000000000000, 5.000000000000000000, 2.000000000000001776 ) ) ;
#18589=FACE_OUTER_BOUND ( 'NONE', #4190, .T. ) ;
#18590=EDGE_CURVE ( 'NONE', #36560, #21953, #40677, .T. ) ;
#18594=EDGE_CURVE ( 'NONE', #46320, #35107, #61924, .T. ) ;
#18596=CARTESIAN_POINT ( 'NONE',  ( -5.000000000000058620, -26.11269837220806522, 2.000000000000001776 ) ) ;
#18604=DIRECTION ( 'NONE',  ( -0.000000000000000000, -1.000000000000000000, -0.000000000000000000 ) ) ;
#18609=LINE ( 'NONE', #7009, #42040 ) ;
#18610=VERTEX_POINT ( 'NONE', #51255 ) ;
#18619=EDGE_LOOP ( 'NONE', ( #47590, #16308, #12317, #11208 ) ) ;
#18624=DIRECTION ( 'NONE',  ( -0.000000000000000000, -0.000000000000000000, -1.000000000000000000 ) ) ;
#18641=VECTOR ( 'NONE', #39015, 1000.000000000000000 ) ;
#18657=DIRECTION ( 'NONE',  ( -1.000000000000000000, 0.000000000000000000, 0.000000000000000000 ) ) ;
#18678=ORIENTED_EDGE ( 'NONE', *, *, #60333, .T. ) ;
#18692=ORIENTED_EDGE ( 'NONE', *, *, #22283, .T. ) ;
#18695=CARTESIAN_POINT ( 'NONE',  ( -36.11269837220801548, 31.11269837220812207, 2.000000000000001776 ) ) ;
#18722=EDGE_LOOP ( 'NONE', ( #7175, #62608, #32869, #31796 ) ) ;
#18729=CARTESIAN_POINT ( 'NONE',  ( -20.55634918610396866, 31.11269837220809009, 2.000000000000000000 ) ) ;
#18752=DIRECTION ( 'NONE',  ( 1.000000000000000000, 0.000000000000000000, 0.000000000000000000 ) ) ;
#18761=EDGE_LOOP ( 'NONE', ( #643, #37887, #885, #27656 ) ) ;
#18763=EDGE_CURVE ( 'NONE', #21301, #13533, #46214, .T. ) ;
#18783=VECTOR ( 'NONE', #51679, 1000.000000000000000 ) ;
#18793=LINE ( 'NONE', #62041, #26239 ) ;
#18811=DIRECTION ( 'NONE',  ( 0.000000000000000000, 0.000000000000000000, 1.000000000000000000 ) ) ;
#18812=LINE ( 'NONE', #56798, #12064 ) ;
#18837=AXIS2_PLACEMENT_3D ( 'NONE', #60022, #17462, #42560 ) ;
#18870=VERTEX_POINT ( 'NONE', #57473 ) ;
#18890=AXIS2_PLACEMENT_3D ( 'NONE', #52843, #63770, #36343 ) ;
#18896=VECTOR ( 'NONE', #31091, 1000.000000000000000 ) ;
#18908=VERTEX_POINT ( 'NONE', #58837 ) ;
#18916=FACE_BOUND ( 'NONE', #46482, .T. ) ;
#18950=ORIENTED_EDGE ( 'NONE', *, *, #30921, .T. ) ;
#18972=EDGE_CURVE ( 'NONE', #21309, #66166, #58162, .T. ) ;
#18988=CIRCLE ( 'NONE', #23513, 72.99999999999998579 ) ;
#19004=DIRECTION ( 'NONE',  ( 0.000000000000000000, -0.000000000000000000, -1.000000000000000000 ) ) ;
#19020=VERTEX_POINT ( 'NONE', #21901 ) ;
#19031=CARTESIAN_POINT ( 'NONE',  ( 2.905661822261151883E-14, 15.55634918610403084, 85.00100000000000477 ) ) ;
#19035=DIRECTION ( 'NONE',  ( -0.000000000000000000, -0.000000000000000000, 1.000000000000000000 ) ) ;
#19049=VERTEX_POINT ( 'NONE', #43349 ) ;
#19050=ORIENTED_EDGE ( 'NONE', *, *, #46516, .F. ) ;
#19061=ORIENTED_EDGE ( 'NONE', *, *, #55592, .T. ) ;
#19070=VERTEX_POINT ( 'NONE', #33165 ) ;
#19093=DIRECTION ( 'NONE',  ( 0.000000000000000000, 0.000000000000000000, 1.000000000000000000 ) ) ;
#19138=AXIS2_PLACEMENT_3D ( 'NONE', #13793, #35251, #8531 ) ;
#19144=ORIENTED_EDGE ( 'NONE', *, *, #49791, .T. ) ;
#19148=ADVANCED_FACE ( 'NONE', ( #57051 ), #24698, .F. ) ;
#19159=LINE ( 'NONE', #67368, #8716 ) ;
#19166=VECTOR ( 'NONE', #10709, 1000.000000000000000 ) ;
#19169=CARTESIAN_POINT ( 'NONE',  ( -20.55634918610396866, 36.11269837220808654, 2.000000000000001776 ) ) ;
#19172=CARTESIAN_POINT ( 'NONE',  ( 10.55634918610397577, -31.11269837220809364, 2.000000000000001776 ) ) ;
#19177=ORIENTED_EDGE ( 'NONE', *, *, #45579, .F. ) ;
#19182=EDGE_CURVE ( 'NONE', #24549, #22892, #67275, .T. ) ;
#19183=CARTESIAN_POINT ( 'NONE',  ( 31.11269837220803325, -15.55634918610409656, 85.00100000000000477 ) ) ;
#19203=DIRECTION ( 'NONE',  ( 0.000000000000000000, 0.000000000000000000, 1.000000000000000000 ) ) ;
#19220=CARTESIAN_POINT ( 'NONE',  ( 0.000000000000000000, 5.000000000000000000, 85.00100000000000477 ) ) ;
#19227=CARTESIAN_POINT ( 'NONE',  ( 2.905661822261151883E-14, 15.55634918610403084, 0.000000000000000000 ) ) ;
#19233=DIRECTION ( 'NONE',  ( -0.000000000000000000, -0.000000000000000000, -1.000000000000000000 ) ) ;
#19246=FACE_BOUND ( 'NONE', #59679, .T. ) ;
#19261=LINE ( 'NONE', #51289, #58746 ) ;
#19270=CARTESIAN_POINT ( 'NONE',  ( 7.762887554996211747E-14, 51.66904755831208718, 2.000000000000001776 ) ) ;
#19283=VERTEX_POINT ( 'NONE', #5977 ) ;
#19294=ADVANCED_FACE ( 'NONE', ( #17229 ), #38704, .F. ) ;
#19296=EDGE_CURVE ( 'NONE', #50609, #4563, #6689, .T. ) ;
#19350=CARTESIAN_POINT ( 'NONE',  ( -46.66904755831212981, -10.55634918610397222, 0.000000000000000000 ) ) ;
#19366=DIRECTION ( 'NONE',  ( -0.000000000000000000, -0.000000000000000000, -1.000000000000000000 ) ) ;
#19369=VERTEX_POINT ( 'NONE', #36115 ) ;
#19375=CARTESIAN_POINT ( 'NONE',  ( -74.99999999999998579, 0.000000000000000000, 85.00000000000000000 ) ) ;
#19380=EDGE_CURVE ( 'NONE', #44589, #13782, #9041, .T. ) ;
#19401=EDGE_CURVE ( 'NONE', #16146, #41880, #3074, .T. ) ;
#19404=ORIENTED_EDGE ( 'NONE', *, *, #28764, .T. ) ;
#19420=FACE_OUTER_BOUND ( 'NONE', #33713, .T. ) ;
#19436=FACE_OUTER_BOUND ( 'NONE', #19796, .T. ) ;
#19451=LINE ( 'NONE', #57095, #104 ) ;
#19459=CARTESIAN_POINT ( 'NONE',  ( -31.11269837220801193, 36.11269837220812207, 85.00100000000000477 ) ) ;
#19464=VECTOR ( 'NONE', #54996, 1000.000000000000000 ) ;
#19481=DIRECTION ( 'NONE',  ( 1.000000000000000000, -0.000000000000000000, 0.000000000000000000 ) ) ;
#19486=VERTEX_POINT ( 'NONE', #16027 ) ;
#19487=ORIENTED_EDGE ( 'NONE', *, *, #62836, .T. ) ;
#19488=AXIS2_PLACEMENT_3D ( 'NONE', #10038, #63167, #30459 ) ;
#19532=ADVANCED_FACE ( 'NONE', ( #16716 ), #4447, .F. ) ;
#19536=LINE ( 'NONE', #3367, #62940 ) ;
#19538=CARTESIAN_POINT ( 'NONE',  ( 46.66904755831207297, -15.55634918610412853, 2.000000000000001776 ) ) ;
#19551=VECTOR ( 'NONE', #63420, 1000.000000000000000 ) ;
#19565=VERTEX_POINT ( 'NONE', #47680 ) ;
#19574=DIRECTION ( 'NONE',  ( 1.000000000000000000, 0.000000000000000000, 0.000000000000000000 ) ) ;
#19593=AXIS2_PLACEMENT_3D ( 'NONE', #33671, #54395, #38581 ) ;
#19609=VERTEX_POINT ( 'NONE', #60683 ) ;
#19646=VECTOR ( 'NONE', #36400, 1000.000000000000000 ) ;
#19667=DIRECTION ( 'NONE',  ( -0.000000000000000000, -1.000000000000000000, -0.000000000000000000 ) ) ;
#19686=VECTOR ( 'NONE', #5164, 1000.000000000000000 ) ;
#19691=ORIENTED_EDGE ( 'NONE', *, *, #41605, .T. ) ;
#19692=DIRECTION ( 'NONE',  ( 0.000000000000000000, -1.000000000000000000, 0.000000000000000000 ) ) ;
#19694=ORIENTED_EDGE ( 'NONE', *, *, #67031, .F. ) ;
#19696=CARTESIAN_POINT ( 'NONE',  ( -51.66904755831212981, -15.55634918610397222, 85.00100000000000477 ) ) ;
#19701=LINE ( 'NONE', #25343, #38879 ) ;
#19730=CARTESIAN_POINT ( 'NONE',  ( -36.11269837220804391, 20.55634918610409301, 2.000000000000001776 ) ) ;
#19740=ORIENTED_EDGE ( 'NONE', *, *, #54789, .F. ) ;
#19770=EDGE_CURVE ( 'NONE', #59267, #44813, #31110, .T. ) ;
#19774=CARTESIAN_POINT ( 'NONE',  ( 0.000000000000000000, 0.000000000000000000, 85.00000000000000000 ) ) ;
#19780=ORIENTED_EDGE ( 'NONE', *, *, #12054, .F. ) ;
#19785=LINE ( 'NONE', #41247, #17514 ) ;
#19796=EDGE_LOOP ( 'NONE', ( #18467, #45686, #4130, #58678 ) ) ;
#19803=CARTESIAN_POINT ( 'NONE',  ( 10.55634918610396511, -46.66904755831214402, 0.000000000000000000 ) ) ;
#19845=EDGE_CURVE ( 'NONE', #41022, #18531, #6781, .T. ) ;
#19849=ORIENTED_EDGE ( 'NONE', *, *, #62963, .T. ) ;
#19868=CARTESIAN_POINT ( 'NONE',  ( -36.11269837220801548, 31.11269837220812207, 0.000000000000000000 ) ) ;
#19871=ORIENTED_EDGE ( 'NONE', *, *, #26539, .F. ) ;
#19893=ORIENTED_EDGE ( 'NONE', *, *, #60815, .F. ) ;
#19895=EDGE_LOOP ( 'NONE', ( #2732, #35229, #2689, #47813 ) ) ;
#19898=LINE ( 'NONE', #41692, #46498 ) ;
#19899=PLANE ( 'NONE',  #64484 ) ;
#19902=AXIS2_PLACEMENT_3D ( 'NONE', #56585, #45335, #62564 ) ;
#19934=EDGE_CURVE ( 'NONE', #58934, #26154, #60156, .T. ) ;
#19942=DIRECTION ( 'NONE',  ( 1.000000000000000000, 0.000000000000000000, 0.000000000000000000 ) ) ;
#19958=FACE_BOUND ( 'NONE', #6502, .T. ) ;
#19963=AXIS2_PLACEMENT_3D ( 'NONE', #41073, #49612, #17621 ) ;
#20025=ADVANCED_FACE ( 'NONE', ( #730 ), #43269, .F. ) ;
#20036=FACE_OUTER_BOUND ( 'NONE', #18446, .T. ) ;
#20049=DIRECTION ( 'NONE',  ( 1.000000000000000000, 0.000000000000000000, 0.000000000000000000 ) ) ;
#20088=EDGE_CURVE ( 'NONE', #65524, #62136, #28144, .T. ) ;
#20101=ORIENTED_EDGE ( 'NONE', *, *, #18594, .T. ) ;
#20102=CARTESIAN_POINT ( 'NONE',  ( 73.43826238111391547, 0.000000000000000000, 26.24939009510892518 ) ) ;
#20109=ORIENTED_EDGE ( 'NONE', *, *, #59984, .T. ) ;
#20114=EDGE_CURVE ( 'NONE', #16433, #47695, #64748, .T. ) ;
#20122=CARTESIAN_POINT ( 'NONE',  ( -54.03875030502680943, 7.289021226777605002E-15, 2.000000000000001776 ) ) ;
#20153=EDGE_LOOP ( 'NONE', ( #42491, #47555, #19177, #45122 ) ) ;
#20154=EDGE_LOOP ( 'NONE', ( #26387, #4613, #65940, #10571 ) ) ;
#20163=DIRECTION ( 'NONE',  ( 0.000000000000000000, 0.000000000000000000, 1.000000000000000000 ) ) ;
#20182=ORIENTED_EDGE ( 'NONE', *, *, #57804, .F. ) ;
#20186=FACE_OUTER_BOUND ( 'NONE', #49621, .T. ) ;
#20214=CARTESIAN_POINT ( 'NONE',  ( 31.11269837220806522, -6.375108774214766072E-14, 2.000000000000001776 ) ) ;
#20228=LINE ( 'NONE', #9331, #5983 ) ;
#20245=CARTESIAN_POINT ( 'NONE',  ( 15.55634918610411610, 46.66904755831205875, 0.000000000000000000 ) ) ;
#20246=DIRECTION ( 'NONE',  ( 1.000000000000000000, 0.000000000000000000, 0.000000000000000000 ) ) ;
#20253=EDGE_CURVE ( 'NONE', #38528, #65730, #57320, .T. ) ;
#20270=CARTESIAN_POINT ( 'NONE',  ( 46.66904755831207297, -15.55634918610412853, 0.000000000000000000 ) ) ;
#20272=CARTESIAN_POINT ( 'NONE',  ( -15.55634918610408945, -31.11269837220804035, 2.000000000000001776 ) ) ;
#20276=LINE ( 'NONE', #29446, #66835 ) ;
#20288=DIRECTION ( 'NONE',  ( -1.000000000000000000, 0.000000000000000000, 0.000000000000000000 ) ) ;
#20297=VECTOR ( 'NONE', #61330, 1000.000000000000000 ) ;
#20329=DIRECTION ( 'NONE',  ( 0.000000000000000000, 1.000000000000000000, -0.000000000000000000 ) ) ;
#20347=ORIENTED_EDGE ( 'NONE', *, *, #58421, .F. ) ;
#20352=DIRECTION ( 'NONE',  ( 1.000000000000000000, -0.000000000000000000, -0.000000000000000000 ) ) ;
#20365=VECTOR ( 'NONE', #63322, 1000.000000000000000 ) ;
#20376=EDGE_LOOP ( 'NONE', ( #9332, #50137, #63981, #48731 ) ) ;
#20389=ORIENTED_EDGE ( 'NONE', *, *, #63127, .T. ) ;
#20440=ORIENTED_EDGE ( 'NONE', *, *, #68411, .F. ) ;
#20445=ORIENTED_EDGE ( 'NONE', *, *, #45032, .T. ) ;
#20447=ADVANCED_FACE ( 'NONE', ( #55140 ), #16125, .F. ) ;
#20462=FACE_OUTER_BOUND ( 'NONE', #26175, .T. ) ;
#20478=DIRECTION ( 'NONE',  ( 0.000000000000000000, 0.000000000000000000, 1.000000000000000000 ) ) ;
#20481=CARTESIAN_POINT ( 'NONE',  ( -15.55634918610411077, -41.66904755831209428, 2.000000000000001776 ) ) ;
#20485=CARTESIAN_POINT ( 'NONE',  ( 31.11269837220809364, 20.55634918610396866, 2.000000000000001776 ) ) ;
#20498=PLANE ( 'NONE',  #18890 ) ;
#20500=AXIS2_PLACEMENT_3D ( 'NONE', #41062, #20288, #30502 ) ;
#20510=LINE ( 'NONE', #69032, #20654 ) ;
#20521=CARTESIAN_POINT ( 'NONE',  ( -5.767955557622883589E-14, -26.11269837220806522, 85.00100000000000477 ) ) ;
#20531=DIRECTION ( 'NONE',  ( 0.000000000000000000, -1.000000000000000000, 0.000000000000000000 ) ) ;
#20534=CARTESIAN_POINT ( 'NONE',  ( 7.762887554996211747E-14, 46.66904755831208718, 2.000000000000001776 ) ) ;
#20553=VECTOR ( 'NONE', #30303, 1000.000000000000000 ) ;
#20555=EDGE_LOOP ( 'NONE', ( #31678, #53853, #57976, #67186 ) ) ;
#20557=ADVANCED_FACE ( 'NONE', ( #2735, #24202, #66080, #17872, #62157, #67457, #3426, #19246, #7676, #35087, #40701, #51617, #39330, #60771, #45645, #2391, #12597, #34052, #66773, #55493, #34755, #7325, #28780, #18564, #40018, #8007, #67124, #18916, #19958, #9053, #14332, #57588, #68151, #32484, #36128, #5738 ), #4464, .F. ) ;
#20569=ORIENTED_EDGE ( 'NONE', *, *, #15242, .T. ) ;
#20571=DIRECTION ( 'NONE',  ( 0.000000000000000000, 1.000000000000000000, -0.000000000000000000 ) ) ;
#20578=ADVANCED_FACE ( 'NONE', ( #20625 ), #31206, .F. ) ;
#20622=LINE ( 'NONE', #42085, #34332 ) ;
#20624=DIRECTION ( 'NONE',  ( 0.000000000000000000, 1.000000000000000000, -0.000000000000000000 ) ) ;
#20625=FACE_OUTER_BOUND ( 'NONE', #22316, .T. ) ;
#20629=ADVANCED_FACE ( 'NONE', ( #3767 ), #41411, .F. ) ;
#20630=ADVANCED_FACE ( 'NONE', ( #36473 ), #57927, .F. ) ;
#20654=VECTOR ( 'NONE', #63785, 1000.000000000000000 ) ;
#20656=ORIENTED_EDGE ( 'NONE', *, *, #51955, .T. ) ;
#20685=DIRECTION ( 'NONE',  ( 0.000000000000000000, -1.000000000000000000, 0.000000000000000000 ) ) ;
#20694=ORIENTED_EDGE ( 'NONE', *, *, #45759, .T. ) ;
#20696=FACE_OUTER_BOUND ( 'NONE', #18082, .T. ) ;
#20717=CARTESIAN_POINT ( 'NONE',  ( -5.000000000000026645, -15.55634918610403616, 85.00100000000000477 ) ) ;
#20722=EDGE_CURVE ( 'NONE', #54708, #12059, #35881, .T. ) ;
#20735=LINE ( 'NONE', #42192, #25687 ) ;
#20737=CARTESIAN_POINT ( 'NONE',  ( -4.999999999999922728, 46.66904755831208718, 2.000000000000000000 ) ) ;
#20740=CARTESIAN_POINT ( 'NONE',  ( -31.11269837220812207, -31.11269837220801193, 85.00100000000000477 ) ) ;
#20756=ADVANCED_FACE ( 'NONE', ( #3518 ), #67900, .F. ) ;
#20809=EDGE_CURVE ( 'NONE', #25475, #33258, #26701, .T. ) ;
#20827=DIRECTION ( 'NONE',  ( -1.000000000000000000, 0.000000000000000000, 0.000000000000000000 ) ) ;
#20843=CARTESIAN_POINT ( 'NONE',  ( 15.55634918610403261, -3.079134169858832593E-14, 0.000000000000000000 ) ) ;
#20860=EDGE_LOOP ( 'NONE', ( #31174, #15858, #11109, #49182 ) ) ;
#20872=ORIENTED_EDGE ( 'NONE', *, *, #13906, .T. ) ;
#20874=LINE ( 'NONE', #42333, #16429 ) ;
#20875=ADVANCED_FACE ( 'NONE', ( #64679 ), #43550, .F. ) ;
#20887=ORIENTED_EDGE ( 'NONE', *, *, #12473, .T. ) ;
#20900=VECTOR ( 'NONE', #62759, 1000.000000000000000 ) ;
#20913=EDGE_LOOP ( 'NONE', ( #55879, #67851, #35947, #26878 ) ) ;
#20941=EDGE_CURVE ( 'NONE', #60552, #65236, #56204, .T. ) ;
#20943=ORIENTED_EDGE ( 'NONE', *, *, #29255, .T. ) ;
#20952=AXIS2_PLACEMENT_3D ( 'NONE', #52522, #58149, #63777 ) ;
#20975=CARTESIAN_POINT ( 'NONE',  ( 31.11269837220812562, 31.11269837220800483, 2.000000000000001776 ) ) ;
#20986=DIRECTION ( 'NONE',  ( -0.000000000000000000, -1.000000000000000000, -0.000000000000000000 ) ) ;
#21057=CARTESIAN_POINT ( 'NONE',  ( 31.11269837220809364, 20.55634918610396866, 0.000000000000000000 ) ) ;
#21059=ORIENTED_EDGE ( 'NONE', *, *, #47316, .F. ) ;
#21060=VECTOR ( 'NONE', #10932, 1000.000000000000000 ) ;
#21069=ORIENTED_EDGE ( 'NONE', *, *, #45579, .T. ) ;
#21076=ADVANCED_FACE ( 'NONE', ( #24564 ), #4476, .F. ) ;
#21090=AXIS2_PLACEMENT_3D ( 'NONE', #30067, #57143, #14568 ) ;
#21097=DIRECTION ( 'NONE',  ( -0.000000000000000000, -0.000000000000000000, -1.000000000000000000 ) ) ;
#21113=ORIENTED_EDGE ( 'NONE', *, *, #22875, .F. ) ;
#21122=VERTEX_POINT ( 'NONE', #68164 ) ;
#21123=ORIENTED_EDGE ( 'NONE', *, *, #23233, .T. ) ;
#21126=CARTESIAN_POINT ( 'NONE',  ( -36.11269837220809364, -10.55634918610397932, 2.000000000000001776 ) ) ;
#21148=ORIENTED_EDGE ( 'NONE', *, *, #4327, .F. ) ;
#21165=PLANE ( 'NONE',  #35418 ) ;
#21168=CARTESIAN_POINT ( 'NONE',  ( -20.55634918610408945, -31.11269837220804035, 85.00100000000000477 ) ) ;
#21210=EDGE_CURVE ( 'NONE', #65730, #16433, #19261, .T. ) ;
#21228=EDGE_LOOP ( 'NONE', ( #40945, #53294, #30734, #29017 ) ) ;
#21263=ORIENTED_EDGE ( 'NONE', *, *, #23846, .T. ) ;
#21268=ADVANCED_FACE ( 'NONE', ( #64250 ), #37167, .F. ) ;
#21301=VERTEX_POINT ( 'NONE', #43128 ) ;
#21309=VERTEX_POINT ( 'NONE', #54370 ) ;
#21310=ORIENTED_EDGE ( 'NONE', *, *, #26122, .T. ) ;
#21312=FACE_BOUND ( 'NONE', #9365, .T. ) ;
#21316=ORIENTED_EDGE ( 'NONE', *, *, #19770, .F. ) ;
#21318=AXIS2_PLACEMENT_3D ( 'NONE', #54018, #60004, #38559 ) ;
#21354=DIRECTION ( 'NONE',  ( -1.000000000000000000, 0.000000000000000000, 0.000000000000000000 ) ) ;
#21360=DIRECTION ( 'NONE',  ( 1.000000000000000000, -0.000000000000000000, 0.000000000000000000 ) ) ;
#21383=DIRECTION ( 'NONE',  ( 1.000000000000000000, -0.000000000000000000, 0.000000000000000000 ) ) ;
#21388=ORIENTED_EDGE ( 'NONE', *, *, #50363, .T. ) ;
#21393=LINE ( 'NONE', #63964, #8115 ) ;
#21413=CARTESIAN_POINT ( 'NONE',  ( -36.11269837220801548, 31.11269837220812207, 85.00100000000000477 ) ) ;
#21421=DIRECTION ( 'NONE',  ( 0.000000000000000000, -0.000000000000000000, -1.000000000000000000 ) ) ;
#21431=CARTESIAN_POINT ( 'NONE',  ( -20.55634918610411077, -41.66904755831209428, 85.00100000000000477 ) ) ;
#21436=DIRECTION ( 'NONE',  ( 0.000000000000000000, -1.000000000000000000, 0.000000000000000000 ) ) ;
#21447=ORIENTED_EDGE ( 'NONE', *, *, #64711, .T. ) ;
#21461=ORIENTED_EDGE ( 'NONE', *, *, #7661, .T. ) ;
#21464=DIRECTION ( 'NONE',  ( -0.000000000000000000, -0.000000000000000000, 1.000000000000000000 ) ) ;
#21478=ORIENTED_EDGE ( 'NONE', *, *, #31218, .F. ) ;
#21485=CARTESIAN_POINT ( 'NONE',  ( 31.11269837220809364, 15.55634918610396866, 2.000000000000001776 ) ) ;
#21491=DIRECTION ( 'NONE',  ( -1.000000000000000000, 0.000000000000000000, 0.000000000000000000 ) ) ;
#21492=DIRECTION ( 'NONE',  ( 0.000000000000000000, 0.000000000000000000, -1.000000000000000000 ) ) ;
#21498=CARTESIAN_POINT ( 'NONE',  ( -46.66904755831212981, -10.55634918610397222, 2.000000000000001776 ) ) ;
#21506=EDGE_LOOP ( 'NONE', ( #56840, #37913, #65256, #5715 ) ) ;
#21520=DIRECTION ( 'NONE',  ( -0.000000000000000000, -0.000000000000000000, -1.000000000000000000 ) ) ;
#21544=LINE ( 'NONE', #32804, #36577 ) ;
#21570=CARTESIAN_POINT ( 'NONE',  ( 0.000000000000000000, 0.000000000000000000, 15.70156211871650775 ) ) ;
#21573=FACE_OUTER_BOUND ( 'NONE', #52217, .T. ) ;
#21580=CARTESIAN_POINT ( 'NONE',  ( -2.645453300864630819E-14, -15.55634918610403616, 2.000000000000001776 ) ) ;
#21612=DIRECTION ( 'NONE',  ( 0.000000000000000000, 1.000000000000000000, 0.000000000000000000 ) ) ;
#21639=ORIENTED_EDGE ( 'NONE', *, *, #41118, .T. ) ;
#21643=DIRECTION ( 'NONE',  ( 0.000000000000000000, -1.000000000000000000, 0.000000000000000000 ) ) ;
#21644=VECTOR ( 'NONE', #27096, 1000.000000000000000 ) ;
#21649=DIRECTION ( 'NONE',  ( 1.000000000000000000, -0.000000000000000000, -0.000000000000000000 ) ) ;
#21664=VECTOR ( 'NONE', #57595, 1000.000000000000000 ) ;
#21667=FACE_OUTER_BOUND ( 'NONE', #2172, .T. ) ;
#21695=VECTOR ( 'NONE', #60708, 1000.000000000000000 ) ;
#21710=VECTOR ( 'NONE', #12467, 1000.000000000000000 ) ;
#21726=PLANE ( 'NONE',  #47401 ) ;
#21746=VECTOR ( 'NONE', #61753, 1000.000000000000000 ) ;
#21811=ORIENTED_EDGE ( 'NONE', *, *, #20253, .T. ) ;
#21821=LINE ( 'NONE', #11612, #9078 ) ;
#21835=EDGE_LOOP ( 'NONE', ( #2570, #25230, #58477, #9664 ) ) ;
#21847=AXIS2_PLACEMENT_3D ( 'NONE', #22051, #949, #28020 ) ;
#21857=EDGE_LOOP ( 'NONE', ( #11340, #20887, #43946, #16847 ) ) ;
#21892=DIRECTION ( 'NONE',  ( 1.000000000000000000, 0.000000000000000000, 0.000000000000000000 ) ) ;
#21894=VECTOR ( 'NONE', #66003, 1000.000000000000000 ) ;
#21901=CARTESIAN_POINT ( 'NONE',  ( 46.66904755831210139, -9.150666335777657423E-14, 2.000000000000001776 ) ) ;
#21920=CARTESIAN_POINT ( 'NONE',  ( -31.11269837220804035, 20.55634918610408945, 0.000000000000000000 ) ) ;
#21939=ORIENTED_EDGE ( 'NONE', *, *, #24011, .T. ) ;
#21953=VERTEX_POINT ( 'NONE', #12273 ) ;
#21979=VERTEX_POINT ( 'NONE', #40389 ) ;
#21986=ORIENTED_EDGE ( 'NONE', *, *, #50807, .T. ) ;
#22007=ORIENTED_EDGE ( 'NONE', *, *, #29255, .F. ) ;
#22008=FACE_OUTER_BOUND ( 'NONE', #49315, .T. ) ;
#22010=FACE_BOUND ( 'NONE', #49744, .T. ) ;
#22012=CARTESIAN_POINT ( 'NONE',  ( 15.55634918610397399, -26.11269837220809364, 0.000000000000000000 ) ) ;
#22023=CARTESIAN_POINT ( 'NONE',  ( 10.55634918610396511, -41.66904755831214402, 0.000000000000000000 ) ) ;
#22040=VECTOR ( 'NONE', #51795, 1000.000000000000000 ) ;
#22051=CARTESIAN_POINT ( 'NONE',  ( 46.66904755831210139, 4.999999999999909406, 85.00100000000000477 ) ) ;
#22061=CARTESIAN_POINT ( 'NONE',  ( -31.11269837220806878, 5.000000000000056843, 2.000000000000001776 ) ) ;
#22072=ORIENTED_EDGE ( 'NONE', *, *, #14830, .T. ) ;
#22086=ORIENTED_EDGE ( 'NONE', *, *, #38328, .T. ) ;
#22090=VECTOR ( 'NONE', #31305, 1000.000000000000000 ) ;
#22092=CARTESIAN_POINT ( 'NONE',  ( 15.55634918610397399, -31.11269837220809364, 0.000000000000000000 ) ) ;
#22095=VERTEX_POINT ( 'NONE', #4151 ) ;
#22111=DIRECTION ( 'NONE',  ( 0.000000000000000000, -0.000000000000000000, -1.000000000000000000 ) ) ;
#22128=FACE_OUTER_BOUND ( 'NONE', #16664, .T. ) ;
#22129=LINE ( 'NONE', #43917, #62954 ) ;
#22143=LINE ( 'NONE', #56495, #25238 ) ;
#22147=EDGE_CURVE ( 'NONE', #33627, #36947, #31233, .T. ) ;
#22157=VECTOR ( 'NONE', #1203, 1000.000000000000000 ) ;
#22166=DIRECTION ( 'NONE',  ( -1.000000000000000000, 0.000000000000000000, 0.000000000000000000 ) ) ;
#22182=VECTOR ( 'NONE', #36965, 1000.000000000000000 ) ;
#22189=CARTESIAN_POINT ( 'NONE',  ( -31.11269837220806878, 5.594483210025202879E-14, 2.000000000000001776 ) ) ;
#22202=ADVANCED_FACE ( 'NONE', ( #25950 ), #36500, .F. ) ;
#22204=DIRECTION ( 'NONE',  ( 0.000000000000000000, 0.000000000000000000, -1.000000000000000000 ) ) ;
#22213=ORIENTED_EDGE ( 'NONE', *, *, #63914, .T. ) ;
#22261=DIRECTION ( 'NONE',  ( -0.000000000000000000, -0.000000000000000000, -1.000000000000000000 ) ) ;
#22276=DIRECTION ( 'NONE',  ( 0.000000000000000000, -0.000000000000000000, -1.000000000000000000 ) ) ;
#22277=ORIENTED_EDGE ( 'NONE', *, *, #42588, .F. ) ;
#22283=EDGE_CURVE ( 'NONE', #11106, #61270, #37525, .T. ) ;
#22313=EDGE_CURVE ( 'NONE', #30419, #22638, #12900, .T. ) ;
#22316=EDGE_LOOP ( 'NONE', ( #44411, #16452, #18556, #44029 ) ) ;
#22331=DIRECTION ( 'NONE',  ( 0.000000000000000000, -1.000000000000000000, 0.000000000000000000 ) ) ;
#22336=ORIENTED_EDGE ( 'NONE', *, *, #7662, .T. ) ;
#22337=EDGE_CURVE ( 'NONE', #16958, #19609, #13244, .T. ) ;
#22344=EDGE_LOOP ( 'NONE', ( #13144, #42346, #23081, #26329 ) ) ;
#22358=CARTESIAN_POINT ( 'NONE',  ( 26.11269837220812562, 31.11269837220800483, 2.000000000000001776 ) ) ;
#22368=FACE_OUTER_BOUND ( 'NONE', #34893, .T. ) ;
#22398=CARTESIAN_POINT ( 'NONE',  ( 74.99999999999998579, 9.184850993605147156E-15, 85.00000000000000000 ) ) ;
#22399=CIRCLE ( 'NONE', #13424, 65.00000000000000000 ) ;
#22401=CARTESIAN_POINT ( 'NONE',  ( 46.66904755831210139, 4.999999999999909406, 0.000000000000000000 ) ) ;
#22403=VERTEX_POINT ( 'NONE', #24145 ) ;
#22419=ORIENTED_EDGE ( 'NONE', *, *, #45581, .F. ) ;
#22441=ORIENTED_EDGE ( 'NONE', *, *, #26379, .F. ) ;
#22450=LINE ( 'NONE', #12600, #62320 ) ;
#22451=ADVANCED_FACE ( 'NONE', ( #56843 ), #19899, .F. ) ;
#22459=CARTESIAN_POINT ( 'NONE',  ( -2.645453300864630819E-14, -15.55634918610403616, 2.000000000000001776 ) ) ;
#22484=CARTESIAN_POINT ( 'NONE',  ( 2.905661822261151883E-14, 20.55634918610402906, 2.000000000000001776 ) ) ;
#22499=EDGE_LOOP ( 'NONE', ( #10703, #1544, #14529, #51698 ) ) ;
#22505=CARTESIAN_POINT ( 'NONE',  ( 15.55634918610411610, 51.66904755831205875, 0.000000000000000000 ) ) ;
#22520=ORIENTED_EDGE ( 'NONE', *, *, #60033, .T. ) ;
#22522=EDGE_LOOP ( 'NONE', ( #63538, #43447, #13532, #14674 ) ) ;
#22572=DIRECTION ( 'NONE',  ( 0.000000000000000000, 1.000000000000000000, 0.000000000000000000 ) ) ;
#22579=LINE ( 'NONE', #33498, #28556 ) ;
#22592=LINE ( 'NONE', #12393, #54326 ) ;
#22607=ORIENTED_EDGE ( 'NONE', *, *, #15404, .F. ) ;
#22627=EDGE_CURVE ( 'NONE', #22403, #66816, #25104, .T. ) ;
#22632=DIRECTION ( 'NONE',  ( -0.000000000000000000, -0.000000000000000000, -1.000000000000000000 ) ) ;
#22633=CARTESIAN_POINT ( 'NONE',  ( -46.66904755831210139, 6.635317295611287136E-14, 85.00100000000000477 ) ) ;
#22638=VERTEX_POINT ( 'NONE', #68013 ) ;
#22644=( NAMED_UNIT ( * ) SI_UNIT ( $, .STERADIAN. ) SOLID_ANGLE_UNIT ( ) );
#22675=LINE ( 'NONE', #11069, #29346 ) ;
#22677=DIRECTION ( 'NONE',  ( -0.000000000000000000, -0.000000000000000000, -1.000000000000000000 ) ) ;
#22693=LINE ( 'NONE', #544, #14282 ) ;
#22702=FACE_BOUND ( 'NONE', #45968, .T. ) ;
#22704=EDGE_CURVE ( 'NONE', #28859, #54708, #69375, .T. ) ;
#22713=VECTOR ( 'NONE', #38009, 1000.000000000000000 ) ;
#22715=DIRECTION ( 'NONE',  ( 0.000000000000000000, 0.000000000000000000, 1.000000000000000000 ) ) ;
#22746=DIRECTION ( 'NONE',  ( 0.000000000000000000, 1.000000000000000000, -0.000000000000000000 ) ) ;
#22769=LINE ( 'NONE', #18541, #69534 ) ;
#22782=EDGE_CURVE ( 'NONE', #13713, #62027, #42305, .T. ) ;
#22786=ADVANCED_FACE ( 'NONE', ( #33497 ), #60903, .F. ) ;
#22789=LINE ( 'NONE', #44593, #36093 ) ;
#22805=ORIENTED_EDGE ( 'NONE', *, *, #43805, .T. ) ;
#22830=VECTOR ( 'NONE', #6560, 1000.000000000000000 ) ;
#22833=ORIENTED_EDGE ( 'NONE', *, *, #28376, .T. ) ;
#22846=ORIENTED_EDGE ( 'NONE', *, *, #54150, .T. ) ;
#22868=VERTEX_POINT ( 'NONE', #8493 ) ;
#22875=EDGE_CURVE ( 'NONE', #56265, #7572, #58852, .T. ) ;
#22876=ORIENTED_EDGE ( 'NONE', *, *, #7740, .T. ) ;
#22878=DIRECTION ( 'NONE',  ( -1.000000000000000000, 0.000000000000000000, 0.000000000000000000 ) ) ;
#22892=VERTEX_POINT ( 'NONE', #19730 ) ;
#22914=LINE ( 'NONE', #33819, #40132 ) ;
#22922=EDGE_LOOP ( 'NONE', ( #36265, #6678, #49644, #23341 ) ) ;
#22942=ADVANCED_FACE ( 'NONE', ( #2519 ), #46452, .F. ) ;
#22968=CARTESIAN_POINT ( 'NONE',  ( 31.11269837220812562, 36.11269837220800838, 85.00100000000000477 ) ) ;
#22972=VECTOR ( 'NONE', #21520, 1000.000000000000000 ) ;
#22981=DIRECTION ( 'NONE',  ( 0.000000000000000000, 1.000000000000000000, -0.000000000000000000 ) ) ;
#22983=VERTEX_POINT ( 'NONE', #62652 ) ;
#23017=VECTOR ( 'NONE', #26982, 1000.000000000000000 ) ;
#23032=VERTEX_POINT ( 'NONE', #9180 ) ;
#23034=CARTESIAN_POINT ( 'NONE',  ( -31.11269837220812207, -26.11269837220801193, 2.000000000000001776 ) ) ;
#23036=CARTESIAN_POINT ( 'NONE',  ( -31.11269837220809364, -15.55634918610397754, 85.00100000000000477 ) ) ;
#23047=DIRECTION ( 'NONE',  ( 0.000000000000000000, -1.000000000000000000, 0.000000000000000000 ) ) ;
#23078=VECTOR ( 'NONE', #48999, 1000.000000000000000 ) ;
#23081=ORIENTED_EDGE ( 'NONE', *, *, #46393, .F. ) ;
#23085=CARTESIAN_POINT ( 'NONE',  ( -31.11269837220809364, -10.55634918610397932, 0.000000000000000000 ) ) ;
#23098=DIRECTION ( 'NONE',  ( -1.000000000000000000, 0.000000000000000000, 0.000000000000000000 ) ) ;
#23105=LINE ( 'NONE', #22401, #2345 ) ;
#23109=EDGE_CURVE ( 'NONE', #37153, #41430, #41533, .T. ) ;
#23110=CARTESIAN_POINT ( 'NONE',  ( 15.55634918610400241, -10.55634918610406281, 0.000000000000000000 ) ) ;
#23112=EDGE_CURVE ( 'NONE', #3968, #40134, #34882, .T. ) ;
#23138=ADVANCED_FACE ( 'NONE', ( #48499 ), #48163, .F. ) ;
#23140=FACE_OUTER_BOUND ( 'NONE', #20154, .T. ) ;
#23144=VERTEX_POINT ( 'NONE', #15829 ) ;
#23176=VECTOR ( 'NONE', #7767, 1000.000000000000000 ) ;
#23177=VERTEX_POINT ( 'NONE', #42890 ) ;
#23196=CARTESIAN_POINT ( 'NONE',  ( 31.11269837220803325, -15.55634918610409656, 85.00100000000000477 ) ) ;
#23203=EDGE_CURVE ( 'NONE', #64405, #23417, #32362, .T. ) ;
#23215=PRODUCT_DEFINITION_SHAPE ( 'NONE', 'NONE',  #16408 ) ;
#23217=DIRECTION ( 'NONE',  ( 0.000000000000000000, 0.000000000000000000, -1.000000000000000000 ) ) ;
#23233=EDGE_CURVE ( 'NONE', #34620, #23417, #22143, .T. ) ;
#23252=VERTEX_POINT ( 'NONE', #59420 ) ;
#23259=DIRECTION ( 'NONE',  ( -0.000000000000000000, -1.000000000000000000, -0.000000000000000000 ) ) ;
#23262=DIRECTION ( 'NONE',  ( 0.000000000000000000, -1.000000000000000000, 0.000000000000000000 ) ) ;
#23298=DIRECTION ( 'NONE',  ( -1.000000000000000000, 0.000000000000000000, 0.000000000000000000 ) ) ;
#23324=ORIENTED_EDGE ( 'NONE', *, *, #28666, .F. ) ;
#23331=VERTEX_POINT ( 'NONE', #52260 ) ;
#23341=ORIENTED_EDGE ( 'NONE', *, *, #59241, .F. ) ;
#23350=EDGE_CURVE ( 'NONE', #49065, #35107, #25547, .T. ) ;
#23380=UNCERTAINTY_MEASURE_WITH_UNIT (LENGTH_MEASURE( 1.000000000000000082E-05 ), #49026, 'distance_accuracy_value', 'NONE');
#23401=ORIENTED_EDGE ( 'NONE', *, *, #49767, .T. ) ;
#23402=DIRECTION ( 'NONE',  ( 1.000000000000000000, 0.000000000000000000, 0.000000000000000000 ) ) ;
#23414=DIRECTION ( 'NONE',  ( 0.000000000000000000, 1.000000000000000000, 0.000000000000000000 ) ) ;
#23417=VERTEX_POINT ( 'NONE', #52930 ) ;
#23443=CARTESIAN_POINT ( 'NONE',  ( -20.55634918610403261, 2.818925648462311528E-14, 0.000000000000000000 ) ) ;
#23451=ORIENTED_EDGE ( 'NONE', *, *, #10728, .T. ) ;
#23458=DIRECTION ( 'NONE',  ( -0.000000000000000000, -1.000000000000000000, -0.000000000000000000 ) ) ;
#23482=LINE ( 'NONE', #44920, #64981 ) ;
#23496=EDGE_LOOP ( 'NONE', ( #59110, #21123, #4063, #38337 ) ) ;
#23501=CARTESIAN_POINT ( 'NONE',  ( 15.55634918610397399, -26.11269837220809364, 85.00100000000000477 ) ) ;
#23512=ORIENTED_EDGE ( 'NONE', *, *, #24071, .T. ) ;
#23513=AXIS2_PLACEMENT_3D ( 'NONE', #11569, #44280, #43926 ) ;
#23526=ORIENTED_EDGE ( 'NONE', *, *, #29637, .T. ) ;
#23542=DIRECTION ( 'NONE',  ( 1.000000000000000000, -0.000000000000000000, 0.000000000000000000 ) ) ;
#23555=FACE_OUTER_BOUND ( 'NONE', #4314, .T. ) ;
#23564=ORIENTED_EDGE ( 'NONE', *, *, #36051, .T. ) ;
#23566=FACE_OUTER_BOUND ( 'NONE', #65822, .T. ) ;
#23572=EDGE_CURVE ( 'NONE', #61065, #31799, #42939, .T. ) ;
#23582=CARTESIAN_POINT ( 'NONE',  ( 66.50000000000000000, 0.000000000000000000, 85.00000000000000000 ) ) ;
#23588=CARTESIAN_POINT ( 'NONE',  ( -15.55634918610400597, 20.55634918610405748, 0.000000000000000000 ) ) ;
#23592=DIRECTION ( 'NONE',  ( 1.000000000000000000, 0.000000000000000000, 0.000000000000000000 ) ) ;
#23660=ORIENTED_EDGE ( 'NONE', *, *, #31234, .F. ) ;
#23664=DIRECTION ( 'NONE',  ( -0.000000000000000000, -0.000000000000000000, -1.000000000000000000 ) ) ;
#23667=EDGE_CURVE ( 'NONE', #50750, #55179, #18609, .T. ) ;
#23741=DIRECTION ( 'NONE',  ( 0.000000000000000000, 1.000000000000000000, -0.000000000000000000 ) ) ;
#23776=CARTESIAN_POINT ( 'NONE',  ( 31.11269837220803325, -15.55634918610409656, 2.000000000000001776 ) ) ;
#23783=CARTESIAN_POINT ( 'NONE',  ( 0.000000000000000000, 0.000000000000000000, 85.00100000000000477 ) ) ;
#23793=DIRECTION ( 'NONE',  ( -0.000000000000000000, -0.000000000000000000, -1.000000000000000000 ) ) ;
#23803=VERTEX_POINT ( 'NONE', #41793 ) ;
#23822=ADVANCED_FACE ( 'NONE', ( #58638 ), #60028, .F. ) ;
#23824=ADVANCED_FACE ( 'NONE', ( #11484 ), #58988, .F. ) ;
#23846=EDGE_CURVE ( 'NONE', #22892, #8745, #64623, .T. ) ;
#23911=EDGE_CURVE ( 'NONE', #2651, #27095, #53707, .T. ) ;
#23913=EDGE_LOOP ( 'NONE', ( #16135, #60322, #39724, #50168 ) ) ;
#23965=DIRECTION ( 'NONE',  ( 1.000000000000000000, 0.000000000000000000, 0.000000000000000000 ) ) ;
#23967=CARTESIAN_POINT ( 'NONE',  ( -31.11269837220801193, 36.11269837220812207, 0.000000000000000000 ) ) ;
#23970=AXIS2_PLACEMENT_3D ( 'NONE', #66308, #56412, #45512 ) ;
#23985=EDGE_CURVE ( 'NONE', #18138, #57137, #33672, .T. ) ;
#23988=PLANE ( 'NONE',  #59227 ) ;
#23996=EDGE_LOOP ( 'NONE', ( #59455, #7177, #51561, #11394 ) ) ;
#24011=EDGE_CURVE ( 'NONE', #38551, #52273, #40662, .T. ) ;
#24018=CONICAL_SURFACE ( 'NONE', #9458, 73.43826238111391547, 0.6747409422235518539 ) ;
#24037=DIRECTION ( 'NONE',  ( 0.000000000000000000, 0.000000000000000000, -1.000000000000000000 ) ) ;
#24046=VECTOR ( 'NONE', #18604, 1000.000000000000000 ) ;
#24057=PLANE ( 'NONE',  #10259 ) ;
#24071=EDGE_CURVE ( 'NONE', #31978, #67838, #27590, .T. ) ;
#24078=ORIENTED_EDGE ( 'NONE', *, *, #613, .F. ) ;
#24086=AXIS2_PLACEMENT_3D ( 'NONE', #58386, #47831, #10196 ) ;
#24098=CARTESIAN_POINT ( 'NONE',  ( 31.11269837220800127, -31.11269837220812562, 2.000000000000001776 ) ) ;
#24116=EDGE_LOOP ( 'NONE', ( #62046, #4550, #840, #65819 ) ) ;
#24127=VERTEX_POINT ( 'NONE', #5783 ) ;
#24129=DIRECTION ( 'NONE',  ( 0.000000000000000000, 1.000000000000000000, 0.000000000000000000 ) ) ;
#24137=VERTEX_POINT ( 'NONE', #53622 ) ;
#24145=CARTESIAN_POINT ( 'NONE',  ( 66.50000000000000000, 0.000000000000000000, 17.57656211871651308 ) ) ;
#24155=DIRECTION ( 'NONE',  ( -0.000000000000000000, -0.000000000000000000, -1.000000000000000000 ) ) ;
#24164=ORIENTED_EDGE ( 'NONE', *, *, #53812, .F. ) ;
#24202=FACE_BOUND ( 'NONE', #28138, .T. ) ;
#24211=ORIENTED_EDGE ( 'NONE', *, *, #66970, .F. ) ;
#24214=PLANE ( 'NONE',  #55798 ) ;
#24218=LINE ( 'NONE', #29828, #66580 ) ;
#24230=PLANE ( 'NONE',  #26518 ) ;
#24236=VECTOR ( 'NONE', #28550, 1000.000000000000000 ) ;
#24240=FACE_OUTER_BOUND ( 'NONE', #61730, .T. ) ;
#24248=AXIS2_PLACEMENT_3D ( 'NONE', #13890, #8967, #3677 ) ;
#24268=LINE ( 'NONE', #46742, #2701 ) ;
#24272=EDGE_LOOP ( 'NONE', ( #42846, #22520, #44832, #67309 ) ) ;
#24273=VECTOR ( 'NONE', #10678, 1000.000000000000000 ) ;
#24284=ORIENTED_EDGE ( 'NONE', *, *, #5851, .F. ) ;
#24322=DIRECTION ( 'NONE',  ( 0.000000000000000000, 0.000000000000000000, -1.000000000000000000 ) ) ;
#24342=ORIENTED_EDGE ( 'NONE', *, *, #64407, .T. ) ;
#24343=VECTOR ( 'NONE', #52421, 1000.000000000000000 ) ;
#24348=DIRECTION ( 'NONE',  ( 0.000000000000000000, 1.000000000000000000, -0.000000000000000000 ) ) ;
#24364=FACE_OUTER_BOUND ( 'NONE', #48427, .T. ) ;
#24384=FACE_OUTER_BOUND ( 'NONE', #14453, .T. ) ;
#24395=ORIENTED_EDGE ( 'NONE', *, *, #30475, .F. ) ;
#24417=CARTESIAN_POINT ( 'NONE',  ( -46.66904755831212981, -10.55634918610397222, 85.00100000000000477 ) ) ;
#24419=DIRECTION ( 'NONE',  ( -0.000000000000000000, -0.000000000000000000, -1.000000000000000000 ) ) ;
#24432=DIRECTION ( 'NONE',  ( 1.000000000000000000, -0.000000000000000000, -0.000000000000000000 ) ) ;
#24433=DIRECTION ( 'NONE',  ( 0.000000000000000000, 0.000000000000000000, -1.000000000000000000 ) ) ;
#24437=VECTOR ( 'NONE', #17503, 1000.000000000000000 ) ;
#24483=DIRECTION ( 'NONE',  ( 0.000000000000000000, 0.000000000000000000, 1.000000000000000000 ) ) ;
#24488=VECTOR ( 'NONE', #5990, 999.9999999999998863 ) ;
#24490=LINE ( 'NONE', #67394, #13506 ) ;
#24496=CARTESIAN_POINT ( 'NONE',  ( 15.55634918610411610, 46.66904755831205875, 2.000000000000001776 ) ) ;
#24503=EDGE_CURVE ( 'NONE', #18610, #4596, #18011, .T. ) ;
#24511=FACE_OUTER_BOUND ( 'NONE', #34400, .T. ) ;
#24522=EDGE_LOOP ( 'NONE', ( #11279, #7803, #48029, #35745 ) ) ;
#24530=ORIENTED_EDGE ( 'NONE', *, *, #49839, .T. ) ;
#24536=CARTESIAN_POINT ( 'NONE',  ( -15.55634918610405748, -15.55634918610400774, 0.000000000000000000 ) ) ;
#24549=VERTEX_POINT ( 'NONE', #41802 ) ;
#24564=FACE_OUTER_BOUND ( 'NONE', #39698, .T. ) ;
#24587=ORIENTED_EDGE ( 'NONE', *, *, #46561, .T. ) ;
#24592=CARTESIAN_POINT ( 'NONE',  ( -20.55634918610405748, -15.55634918610400774, 2.000000000000000000 ) ) ;
#24608=DIRECTION ( 'NONE',  ( -1.000000000000000000, 0.000000000000000000, 0.000000000000000000 ) ) ;
#24613=LINE ( 'NONE', #4524, #10348 ) ;
#24636=FACE_OUTER_BOUND ( 'NONE', #32210, .T. ) ;
#24660=LINE ( 'NONE', #1818, #52939 ) ;
#24667=LINE ( 'NONE', #67245, #2704 ) ;
#24670=ORIENTED_EDGE ( 'NONE', *, *, #37323, .F. ) ;
#24690=LINE ( 'NONE', #45437, #44196 ) ;
#24698=PLANE ( 'NONE',  #61975 ) ;
#24708=EDGE_CURVE ( 'NONE', #50424, #50563, #66744, .T. ) ;
#24714=EDGE_LOOP ( 'NONE', ( #23401, #8807, #51355, #13941 ) ) ;
#24715=CARTESIAN_POINT ( 'NONE',  ( -20.55634918610411077, -41.66904755831209428, 0.000000000000000000 ) ) ;
#24769=DIRECTION ( 'NONE',  ( 1.000000000000000000, -0.000000000000000000, -0.000000000000000000 ) ) ;
#24778=EDGE_CURVE ( 'NONE', #68402, #54490, #56866, .T. ) ;
#24811=CARTESIAN_POINT ( 'NONE',  ( 31.11269837220806522, -6.375108774214766072E-14, 85.00100000000000477 ) ) ;
#24851=AXIS2_PLACEMENT_3D ( 'NONE', #15716, #31219, #43125 ) ;
#24874=ORIENTED_EDGE ( 'NONE', *, *, #37228, .T. ) ;
#24877=EDGE_LOOP ( 'NONE', ( #37818, #63812, #44840, #57526 ) ) ;
#24890=ORIENTED_EDGE ( 'NONE', *, *, #46085, .T. ) ;
#24901=VECTOR ( 'NONE', #42290, 1000.000000000000000 ) ;
#24912=ORIENTED_EDGE ( 'NONE', *, *, #15247, .T. ) ;
#24914=ORIENTED_EDGE ( 'NONE', *, *, #33696, .F. ) ;
#24923=ORIENTED_EDGE ( 'NONE', *, *, #62429, .F. ) ;
#24925=ORIENTED_EDGE ( 'NONE', *, *, #1009, .T. ) ;
#24929=VERTEX_POINT ( 'NONE', #16006 ) ;
#24944=EDGE_CURVE ( 'NONE', #5719, #30890, #38506, .T. ) ;
#24978=LINE ( 'NONE', #42767, #14390 ) ;
#24983=CARTESIAN_POINT ( 'NONE',  ( 26.11269837220800127, -31.11269837220812562, 0.000000000000000000 ) ) ;
#25006=CARTESIAN_POINT ( 'NONE',  ( -51.66904755831212981, -10.55634918610397222, 85.00100000000000477 ) ) ;
#25013=ORIENTED_EDGE ( 'NONE', *, *, #45188, .T. ) ;
#25016=LINE ( 'NONE', #3216, #69238 ) ;
#25020=DIRECTION ( 'NONE',  ( 1.000000000000000000, 0.000000000000000000, 0.000000000000000000 ) ) ;
#25041=AXIS2_PLACEMENT_3D ( 'NONE', #25237, #46675, #9743 ) ;
#25045=EDGE_LOOP ( 'NONE', ( #41482, #58863, #31310, #40439 ) ) ;
#25052=ORIENTED_EDGE ( 'NONE', *, *, #26667, .T. ) ;
#25071=PLANE ( 'NONE',  #30112 ) ;
#25087=CARTESIAN_POINT ( 'NONE',  ( -31.11269837220806878, 5.000000000000056843, 85.00100000000000477 ) ) ;
#25092=DIRECTION ( 'NONE',  ( -1.000000000000000000, 0.000000000000000000, 0.000000000000000000 ) ) ;
#25104=LINE ( 'NONE', #9611, #48688 ) ;
#25118=ADVANCED_FACE ( 'NONE', ( #39562 ), #29021, .F. ) ;
#25120=ORIENTED_EDGE ( 'NONE', *, *, #29225, .F. ) ;
#25173=DIRECTION ( 'NONE',  ( -1.000000000000000000, 0.000000000000000000, 0.000000000000000000 ) ) ;
#25176=DIRECTION ( 'NONE',  ( -0.000000000000000000, -0.000000000000000000, -1.000000000000000000 ) ) ;
#25195=ORIENTED_EDGE ( 'NONE', *, *, #46964, .F. ) ;
#25204=AXIS2_PLACEMENT_3D ( 'NONE', #60496, #21464, #64732 ) ;
#25225=DIRECTION ( 'NONE',  ( -0.000000000000000000, -0.000000000000000000, -1.000000000000000000 ) ) ;
#25228=CARTESIAN_POINT ( 'NONE',  ( -36.11269837220809364, -15.55634918610397754, 85.00100000000000477 ) ) ;
#25230=ORIENTED_EDGE ( 'NONE', *, *, #3399, .T. ) ;
#25235=ORIENTED_EDGE ( 'NONE', *, *, #68387, .F. ) ;
#25237=CARTESIAN_POINT ( 'NONE',  ( 41.66904755831212981, 15.55634918610394379, 85.00100000000000477 ) ) ;
#25238=VECTOR ( 'NONE', #8325, 1000.000000000000000 ) ;
#25248=ORIENTED_EDGE ( 'NONE', *, *, #13459, .F. ) ;
#25263=ORIENTED_EDGE ( 'NONE', *, *, #11979, .F. ) ;
#25292=EDGE_CURVE ( 'NONE', #62027, #15785, #59515, .T. ) ;
#25293=EDGE_CURVE ( 'NONE', #5765, #62805, #64462, .T. ) ;
#25306=ORIENTED_EDGE ( 'NONE', *, *, #51572, .T. ) ;
#25311=LINE ( 'NONE', #40090, #13940 ) ;
#25324=ADVANCED_FACE ( 'NONE', ( #69397 ), #63786, .F. ) ;
#25329=VECTOR ( 'NONE', #39410, 1000.000000000000000 ) ;
#25334=ORIENTED_EDGE ( 'NONE', *, *, #52548, .T. ) ;
#25336=CARTESIAN_POINT ( 'NONE',  ( 15.55634918610411610, 51.66904755831205875, 2.000000000000001776 ) ) ;
#25343=CARTESIAN_POINT ( 'NONE',  ( 46.66904755831207297, -15.55634918610412853, 0.000000000000000000 ) ) ;
#25350=EDGE_CURVE ( 'NONE', #42408, #13782, #21544, .T. ) ;
#25352=CARTESIAN_POINT ( 'NONE',  ( 41.66904755831212981, 20.55634918610394379, 0.000000000000000000 ) ) ;
#25356=EDGE_CURVE ( 'NONE', #8504, #66166, #69033, .T. ) ;
#25358=CARTESIAN_POINT ( 'NONE',  ( 26.11269837220806167, -6.375108774214766072E-14, 0.000000000000000000 ) ) ;
#25366=VERTEX_POINT ( 'NONE', #16955 ) ;
#25402=VECTOR ( 'NONE', #7157, 1000.000000000000000 ) ;
#25428=FACE_OUTER_BOUND ( 'NONE', #28709, .T. ) ;
#25439=DIRECTION ( 'NONE',  ( 0.000000000000000000, 0.000000000000000000, -1.000000000000000000 ) ) ;
#25440=VECTOR ( 'NONE', #44732, 1000.000000000000000 ) ;
#25474=CARTESIAN_POINT ( 'NONE',  ( -15.55634918610400597, 20.55634918610405748, 0.000000000000000000 ) ) ;
#25475=VERTEX_POINT ( 'NONE', #34898 ) ;
#25479=VECTOR ( 'NONE', #14348, 1000.000000000000000 ) ;
#25547=LINE ( 'NONE', #41707, #11705 ) ;
#25550=VECTOR ( 'NONE', #43028, 1000.000000000000000 ) ;
#25563=ORIENTED_EDGE ( 'NONE', *, *, #64988, .F. ) ;
#25571=CARTESIAN_POINT ( 'NONE',  ( -15.55634918610411077, -46.66904755831208718, 85.00100000000000477 ) ) ;
#25578=VECTOR ( 'NONE', #33319, 1000.000000000000000 ) ;
#25585=ORIENTED_EDGE ( 'NONE', *, *, #54699, .F. ) ;
#25600=ORIENTED_EDGE ( 'NONE', *, *, #10230, .F. ) ;
#25624=VECTOR ( 'NONE', #32981, 1000.000000000000000 ) ;
#25668=PLANE ( 'NONE',  #46272 ) ;
#25679=CARTESIAN_POINT ( 'NONE',  ( -5.767955557622883589E-14, -31.11269837220806878, 2.000000000000001776 ) ) ;
#25687=VECTOR ( 'NONE', #63656, 1000.000000000000000 ) ;
#25703=DIRECTION ( 'NONE',  ( 1.000000000000000000, 0.000000000000000000, 0.000000000000000000 ) ) ;
#25726=VERTEX_POINT ( 'NONE', #32033 ) ;
#25738=ORIENTED_EDGE ( 'NONE', *, *, #7662, .F. ) ;
#25743=EDGE_LOOP ( 'NONE', ( #67168, #54680, #60983, #6809 ) ) ;
#25776=EDGE_LOOP ( 'NONE', ( #63884, #9604, #44304, #46673 ) ) ;
#25797=CARTESIAN_POINT ( 'NONE',  ( -20.55634918610403261, 2.818925648462311528E-14, 85.00100000000000477 ) ) ;
#25801=CARTESIAN_POINT ( 'NONE',  ( -2.645453300864630819E-14, -15.55634918610403616, 85.00100000000000477 ) ) ;
#25805=CARTESIAN_POINT ( 'NONE',  ( -2.645453300864630819E-14, -15.55634918610403616, 85.00100000000000477 ) ) ;
#25824=DIRECTION ( 'NONE',  ( 0.000000000000000000, 0.000000000000000000, 1.000000000000000000 ) ) ;
#25859=DIRECTION ( 'NONE',  ( 1.000000000000000000, 0.000000000000000000, 0.000000000000000000 ) ) ;
#25862=VECTOR ( 'NONE', #39872, 1000.000000000000000 ) ;
#25866=CARTESIAN_POINT ( 'NONE',  ( -5.767955557622883589E-14, -31.11269837220806878, 2.000000000000001776 ) ) ;
#25887=EDGE_CURVE ( 'NONE', #59151, #36200, #34820, .T. ) ;
#25909=DIRECTION ( 'NONE',  ( -1.000000000000000000, 0.000000000000000000, 0.000000000000000000 ) ) ;
#25910=CARTESIAN_POINT ( 'NONE',  ( 6.375108774214766072E-14, 36.11269837220805812, 85.00100000000000477 ) ) ;
#25920=ORIENTED_EDGE ( 'NONE', *, *, #4208, .T. ) ;
#25925=EDGE_CURVE ( 'NONE', #32583, #28859, #69565, .T. ) ;
#25950=FACE_OUTER_BOUND ( 'NONE', #68490, .T. ) ;
#25959=CARTESIAN_POINT ( 'NONE',  ( -36.11269837220804391, 15.55634918610408945, 85.00100000000000477 ) ) ;
#25960=ORIENTED_EDGE ( 'NONE', *, *, #1192, .T. ) ;
#25975=PLANE ( 'NONE',  #3141 ) ;
#25977=ORIENTED_EDGE ( 'NONE', *, *, #59630, .T. ) ;
#25983=ADVANCED_FACE ( 'NONE', ( #51169 ), #2629, .F. ) ;
#25992=CARTESIAN_POINT ( 'NONE',  ( 6.375108774214766072E-14, 36.11269837220805812, 0.000000000000000000 ) ) ;
#26039=VECTOR ( 'NONE', #52286, 1000.000000000000000 ) ;
#26063=ORIENTED_EDGE ( 'NONE', *, *, #59692, .F. ) ;
#26077=VERTEX_POINT ( 'NONE', #40953 ) ;
#26092=DIRECTION ( 'NONE',  ( 0.000000000000000000, 1.000000000000000000, 0.000000000000000000 ) ) ;
#26096=EDGE_CURVE ( 'NONE', #21122, #21979, #37053, .T. ) ;
#26109=DIRECTION ( 'NONE',  ( 0.000000000000000000, 0.000000000000000000, 1.000000000000000000 ) ) ;
#26122=EDGE_CURVE ( 'NONE', #18870, #51157, #20874, .T. ) ;
#26130=CARTESIAN_POINT ( 'NONE',  ( -36.11269837220801548, 31.11269837220812207, 2.000000000000000000 ) ) ;
#26139=VECTOR ( 'NONE', #18432, 1000.000000000000000 ) ;
#26144=FACE_OUTER_BOUND ( 'NONE', #50341, .T. ) ;
#26148=EDGE_CURVE ( 'NONE', #11547, #62136, #5391, .T. ) ;
#26154=VERTEX_POINT ( 'NONE', #16287 ) ;
#26159=EDGE_LOOP ( 'NONE', ( #52272, #69149, #41528, #37177 ) ) ;
#26160=DIRECTION ( 'NONE',  ( -0.000000000000000000, -0.000000000000000000, -1.000000000000000000 ) ) ;
#26169=FACE_OUTER_BOUND ( 'NONE', #12650, .T. ) ;
#26175=EDGE_LOOP ( 'NONE', ( #60541, #35415, #59872, #54035 ) ) ;
#26208=EDGE_CURVE ( 'NONE', #45426, #16958, #26845, .T. ) ;
#26239=VECTOR ( 'NONE', #24432, 1000.000000000000000 ) ;
#26287=ORIENTED_EDGE ( 'NONE', *, *, #60185, .F. ) ;
#26288=AXIS2_PLACEMENT_3D ( 'NONE', #49577, #6, #48520 ) ;
#26293=VECTOR ( 'NONE', #17590, 1000.000000000000000 ) ;
#26303=AXIS2_PLACEMENT_3D ( 'NONE', #48245, #16254, #26816 ) ;
#26305=ORIENTED_EDGE ( 'NONE', *, *, #69066, .T. ) ;
#26306=LINE ( 'NONE', #40742, #52191 ) ;
#26315=ORIENTED_EDGE ( 'NONE', *, *, #62074, .F. ) ;
#26317=LINE ( 'NONE', #59347, #34079 ) ;
#26329=ORIENTED_EDGE ( 'NONE', *, *, #24708, .F. ) ;
#26330=LINE ( 'NONE', #10140, #43516 ) ;
#26349=ORIENTED_EDGE ( 'NONE', *, *, #3344, .F. ) ;
#26354=EDGE_CURVE ( 'NONE', #8516, #25726, #45450, .T. ) ;
#26379=EDGE_CURVE ( 'NONE', #19049, #53174, #33529, .T. ) ;
#26384=ORIENTED_EDGE ( 'NONE', *, *, #54356, .T. ) ;
#26387=ORIENTED_EDGE ( 'NONE', *, *, #28912, .T. ) ;
#26392=DIRECTION ( 'NONE',  ( -0.000000000000000000, -0.000000000000000000, -1.000000000000000000 ) ) ;
#26393=FACE_OUTER_BOUND ( 'NONE', #15842, .T. ) ;
#26397=ORIENTED_EDGE ( 'NONE', *, *, #58421, .T. ) ;
#26398=EDGE_LOOP ( 'NONE', ( #1482, #37700, #51981, #34010 ) ) ;
#26420=VERTEX_POINT ( 'NONE', #50036 ) ;
#26432=EDGE_CURVE ( 'NONE', #9968, #53834, #55658, .T. ) ;
#26436=EDGE_CURVE ( 'NONE', #30631, #46713, #28941, .T. ) ;
#26443=DIRECTION ( 'NONE',  ( -0.000000000000000000, -1.000000000000000000, -0.000000000000000000 ) ) ;
#26445=CARTESIAN_POINT ( 'NONE',  ( -15.55634918610400597, 15.55634918610405748, 2.000000000000001776 ) ) ;
#26454=ORIENTED_EDGE ( 'NONE', *, *, #52390, .F. ) ;
#26490=DIRECTION ( 'NONE',  ( 0.000000000000000000, 1.000000000000000000, 0.000000000000000000 ) ) ;
#26518=AXIS2_PLACEMENT_3D ( 'NONE', #66455, #67482, #35466 ) ;
#26539=EDGE_CURVE ( 'NONE', #67789, #64323, #57742, .T. ) ;
#26581=EDGE_CURVE ( 'NONE', #10664, #19486, #68632, .T. ) ;
#26597=FACE_BOUND ( 'NONE', #6641, .T. ) ;
#26618=FACE_OUTER_BOUND ( 'NONE', #24877, .T. ) ;
#26628=VECTOR ( 'NONE', #40735, 1000.000000000000000 ) ;
#26632=ORIENTED_EDGE ( 'NONE', *, *, #50604, .T. ) ;
#26637=DIRECTION ( 'NONE',  ( -1.000000000000000000, 0.000000000000000000, 0.000000000000000000 ) ) ;
#26641=LINE ( 'NONE', #17742, #22157 ) ;
#26667=EDGE_CURVE ( 'NONE', #1187, #19020, #62700, .T. ) ;
#26674=CARTESIAN_POINT ( 'NONE',  ( -15.55634918610405748, -15.55634918610400774, 0.000000000000000000 ) ) ;
#26681=VECTOR ( 'NONE', #32929, 1000.000000000000000 ) ;
#26701=LINE ( 'NONE', #22459, #10400 ) ;
#26706=VECTOR ( 'NONE', #49488, 1000.000000000000000 ) ;
#26708=EDGE_CURVE ( 'NONE', #22983, #24137, #26784, .T. ) ;
#26732=CARTESIAN_POINT ( 'NONE',  ( -31.11269837220801193, 31.11269837220812207, 85.00100000000000477 ) ) ;
#26743=DIRECTION ( 'NONE',  ( 0.000000000000000000, 1.000000000000000000, -0.000000000000000000 ) ) ;
#26744=ADVANCED_FACE ( 'NONE', ( #36306 ), #21165, .F. ) ;
#26745=CARTESIAN_POINT ( 'NONE',  ( 46.66904755831212981, 20.55634918610394379, 0.000000000000000000 ) ) ;
#26764=EDGE_CURVE ( 'NONE', #53791, #62932, #42270, .T. ) ;
#26784=LINE ( 'NONE', #36, #28688 ) ;
#26815=PRODUCT_DEFINITION_CONTEXT ( 'detailed design', #59285, 'design' ) ;
#26816=DIRECTION ( 'NONE',  ( 0.000000000000000000, -0.000000000000000000, -1.000000000000000000 ) ) ;
#26830=EDGE_LOOP ( 'NONE', ( #6257, #29472, #37040, #61712 ) ) ;
#26831=FACE_OUTER_BOUND ( 'NONE', #26159, .T. ) ;
#26845=LINE ( 'NONE', #11696, #4096 ) ;
#26878=ORIENTED_EDGE ( 'NONE', *, *, #43017, .T. ) ;
#26889=VERTEX_POINT ( 'NONE', #45391 ) ;
#26921=VERTEX_POINT ( 'NONE', #8108 ) ;
#26929=AXIS2_PLACEMENT_3D ( 'NONE', #54810, #49171, #18233 ) ;
#26935=DIRECTION ( 'NONE',  ( 1.000000000000000000, 0.000000000000000000, 0.000000000000000000 ) ) ;
#26941=VERTEX_POINT ( 'NONE', #19350 ) ;
#26975=CARTESIAN_POINT ( 'NONE',  ( -20.55634918610411077, -46.66904755831208718, 2.000000000000001776 ) ) ;
#26982=DIRECTION ( 'NONE',  ( 0.000000000000000000, -1.000000000000000000, 0.000000000000000000 ) ) ;
#26985=LINE ( 'NONE', #53709, #43324 ) ;
#26986=LINE ( 'NONE', #28027, #17639 ) ;
#26991=EDGE_CURVE ( 'NONE', #47843, #8605, #4555, .T. ) ;
#27038=CARTESIAN_POINT ( 'NONE',  ( 10.55634918610397577, -31.11269837220809364, 85.00100000000000477 ) ) ;
#27039=DIRECTION ( 'NONE',  ( 1.000000000000000000, 0.000000000000000000, 0.000000000000000000 ) ) ;
#27053=ORIENTED_EDGE ( 'NONE', *, *, #2926, .T. ) ;
#27054=CARTESIAN_POINT ( 'NONE',  ( 15.55634918610403261, -3.079134169858832593E-14, 2.000000000000001776 ) ) ;
#27081=VERTEX_POINT ( 'NONE', #65381 ) ;
#27095=VERTEX_POINT ( 'NONE', #35723 ) ;
#27096=DIRECTION ( 'NONE',  ( -0.000000000000000000, -0.000000000000000000, -1.000000000000000000 ) ) ;
#27107=CARTESIAN_POINT ( 'NONE',  ( -31.11269837220806878, 5.594483210025202879E-14, 0.000000000000000000 ) ) ;
#27109=DIRECTION ( 'NONE',  ( 0.000000000000000000, 1.000000000000000000, -0.000000000000000000 ) ) ;
#27113=ORIENTED_EDGE ( 'NONE', *, *, #42588, .T. ) ;
#27149=DIRECTION ( 'NONE',  ( -1.000000000000000000, 0.000000000000000000, 0.000000000000000000 ) ) ;
#27163=CYLINDRICAL_SURFACE ( 'NONE', #45899, 65.00000000000000000 ) ;
#27166=DIRECTION ( 'NONE',  ( -0.000000000000000000, -0.000000000000000000, -1.000000000000000000 ) ) ;
#27167=LINE ( 'NONE', #38426, #39751 ) ;
#27171=ADVANCED_FACE ( 'NONE', ( #33723 ), #57515, .F. ) ;
#27175=VECTOR ( 'NONE', #15968, 1000.000000000000000 ) ;
#27204=EDGE_CURVE ( 'NONE', #33686, #63697, #46603, .T. ) ;
#27210=VERTEX_POINT ( 'NONE', #52576 ) ;
#27217=CARTESIAN_POINT ( 'NONE',  ( -15.55634918610396866, 36.11269837220808654, 85.00100000000000477 ) ) ;
#27221=CARTESIAN_POINT ( 'NONE',  ( -46.66904755831212981, -15.55634918610397222, 2.000000000000001776 ) ) ;
#27235=ORIENTED_EDGE ( 'NONE', *, *, #20114, .F. ) ;
#27245=EDGE_LOOP ( 'NONE', ( #3879, #50922, #4958, #32073 ) ) ;
#27256=ORIENTED_EDGE ( 'NONE', *, *, #44792, .T. ) ;
#27272=DIRECTION ( 'NONE',  ( -0.000000000000000000, -0.000000000000000000, 1.000000000000000000 ) ) ;
#27274=FACE_BOUND ( 'NONE', #51990, .T. ) ;
#27282=CARTESIAN_POINT ( 'NONE',  ( 31.11269837220812562, 31.11269837220800483, 0.000000000000000000 ) ) ;
#27345=ORIENTED_EDGE ( 'NONE', *, *, #5761, .T. ) ;
#27368=EDGE_CURVE ( 'NONE', #67388, #16433, #11379, .T. ) ;
#27387=ORIENTED_EDGE ( 'NONE', *, *, #54850, .T. ) ;
#27388=LINE ( 'NONE', #60095, #16120 ) ;
#27394=CARTESIAN_POINT ( 'NONE',  ( 15.55634918610409656, 36.11269837220803680, 0.000000000000000000 ) ) ;
#27458=LINE ( 'NONE', #34850, #23176 ) ;
#27462=VECTOR ( 'NONE', #21360, 1000.000000000000000 ) ;
#27467=DIRECTION ( 'NONE',  ( 1.000000000000000000, 0.000000000000000000, 0.000000000000000000 ) ) ;
#27469=CARTESIAN_POINT ( 'NONE',  ( 41.66904755831208007, -15.55634918610412853, 2.000000000000001776 ) ) ;
#27529=ORIENTED_EDGE ( 'NONE', *, *, #45169, .F. ) ;
#27564=VECTOR ( 'NONE', #49705, 1000.000000000000000 ) ;
#27565=( LENGTH_UNIT ( ) NAMED_UNIT ( * ) SI_UNIT ( .MILLI., .METRE. ) );
#27571=ADVANCED_FACE ( 'NONE', ( #15209 ), #4995, .F. ) ;
#27586=CARTESIAN_POINT ( 'NONE',  ( 26.11269837220809364, 15.55634918610396866, 0.000000000000000000 ) ) ;
#27590=LINE ( 'NONE', #10716, #37611 ) ;
#27604=CARTESIAN_POINT ( 'NONE',  ( 15.55634918610409656, 31.11269837220803325, 0.000000000000000000 ) ) ;
#27624=VECTOR ( 'NONE', #44334, 1000.000000000000000 ) ;
#27626=CARTESIAN_POINT ( 'NONE',  ( -20.55634918610400419, 15.55634918610405748, 2.000000000000000000 ) ) ;
#27628=DIRECTION ( 'NONE',  ( 1.000000000000000000, 0.000000000000000000, -0.000000000000000000 ) ) ;
#27644=DIRECTION ( 'NONE',  ( 0.000000000000000000, 1.000000000000000000, 0.000000000000000000 ) ) ;
#27649=CARTESIAN_POINT ( 'NONE',  ( -51.66904755831210139, 6.635317295611287136E-14, 0.000000000000000000 ) ) ;
#27656=ORIENTED_EDGE ( 'NONE', *, *, #36703, .F. ) ;
#27664=CARTESIAN_POINT ( 'NONE',  ( 2.905661822261151883E-14, 20.55634918610402906, 2.000000000000001776 ) ) ;
#27694=EDGE_CURVE ( 'NONE', #67865, #27081, #54197, .T. ) ;
#27700=LINE ( 'NONE', #60758, #8329 ) ;
#27748=DIRECTION ( 'NONE',  ( 1.000000000000000000, -0.000000000000000000, 0.000000000000000000 ) ) ;
#27755=ORIENTED_EDGE ( 'NONE', *, *, #61464, .F. ) ;
#27758=ORIENTED_EDGE ( 'NONE', *, *, #64498, .T. ) ;
#27762=VECTOR ( 'NONE', #31921, 1000.000000000000000 ) ;
#27776=VECTOR ( 'NONE', #37961, 1000.000000000000000 ) ;
#27783=CARTESIAN_POINT ( 'NONE',  ( -31.11269837220804035, 15.55634918610408945, 2.000000000000001776 ) ) ;
#27800=DIRECTION ( 'NONE',  ( -0.000000000000000000, -0.000000000000000000, -1.000000000000000000 ) ) ;
#27835=VERTEX_POINT ( 'NONE', #61593 ) ;
#27868=FACE_OUTER_BOUND ( 'NONE', #49295, .T. ) ;
#27874=CARTESIAN_POINT ( 'NONE',  ( -31.11269837220801193, 31.11269837220812207, 0.000000000000000000 ) ) ;
#27886=ORIENTED_EDGE ( 'NONE', *, *, #28862, .T. ) ;
#27902=PLANE ( 'NONE',  #32109 ) ;
#27905=ORIENTED_EDGE ( 'NONE', *, *, #4740, .T. ) ;
#27929=EDGE_CURVE ( 'NONE', #62528, #44589, #65395, .T. ) ;
#27957=VERTEX_POINT ( 'NONE', #16152 ) ;
#27977=FACE_BOUND ( 'NONE', #36095, .T. ) ;
#28014=CARTESIAN_POINT ( 'NONE',  ( 10.55634918610403084, -3.079134169858832593E-14, 85.00100000000000477 ) ) ;
#28020=DIRECTION ( 'NONE',  ( 0.000000000000000000, 0.000000000000000000, 1.000000000000000000 ) ) ;
#28027=CARTESIAN_POINT ( 'NONE',  ( 10.55634918610396511, -46.66904755831214402, 0.000000000000000000 ) ) ;
#28030=EDGE_CURVE ( 'NONE', #4856, #30419, #54821, .T. ) ;
#28037=ADVANCED_FACE ( 'NONE', ( #60460 ), #12274, .F. ) ;
#28049=PLANE ( 'NONE',  #59962 ) ;
#28055=CARTESIAN_POINT ( 'NONE',  ( 15.55634918610411610, 46.66904755831205875, 85.00100000000000477 ) ) ;
#28059=LINE ( 'NONE', #17504, #15840 ) ;
#28073=ORIENTED_EDGE ( 'NONE', *, *, #14607, .F. ) ;
#28101=DIRECTION ( 'NONE',  ( 1.000000000000000000, 0.000000000000000000, 0.000000000000000000 ) ) ;
#28114=ORIENTED_EDGE ( 'NONE', *, *, #22313, .T. ) ;
#28126=ORIENTED_EDGE ( 'NONE', *, *, #23911, .T. ) ;
#28130=FACE_OUTER_BOUND ( 'NONE', #28244, .T. ) ;
#28137=LINE ( 'NONE', #42593, #32847 ) ;
#28138=EDGE_LOOP ( 'NONE', ( #33338, #801, #1106, #29452 ) ) ;
#28144=LINE ( 'NONE', #44686, #46258 ) ;
#28151=LINE ( 'NONE', #16213, #51399 ) ;
#28166=ADVANCED_FACE ( 'NONE', ( #2764 ), #24230, .F. ) ;
#28190=VECTOR ( 'NONE', #2046, 1000.000000000000000 ) ;
#28191=DIRECTION ( 'NONE',  ( -1.000000000000000000, 0.000000000000000000, 0.000000000000000000 ) ) ;
#28203=CARTESIAN_POINT ( 'NONE',  ( -36.11269837220801548, 36.11269837220812207, 85.00100000000000477 ) ) ;
#28244=EDGE_LOOP ( 'NONE', ( #29276, #33899, #54073, #61181 ) ) ;
#28269=ORIENTED_EDGE ( 'NONE', *, *, #45759, .F. ) ;
#28278=AXIS2_PLACEMENT_3D ( 'NONE', #30735, #63083, #4677 ) ;
#28287=AXIS2_PLACEMENT_3D ( 'NONE', #25910, #43100, #42755 ) ;
#28355=LINE ( 'NONE', #61747, #47176 ) ;
#28363=CARTESIAN_POINT ( 'NONE',  ( -5.000000000000058620, -26.11269837220806522, 85.00100000000000477 ) ) ;
#28369=EDGE_CURVE ( 'NONE', #63634, #21301, #11139, .T. ) ;
#28376=EDGE_CURVE ( 'NONE', #19070, #12059, #38937, .T. ) ;
#28383=DIRECTION ( 'NONE',  ( 0.000000000000000000, -1.000000000000000000, 0.000000000000000000 ) ) ;
#28387=ORIENTED_EDGE ( 'NONE', *, *, #16655, .F. ) ;
#28409=CARTESIAN_POINT ( 'NONE',  ( 26.11269837220800127, -31.11269837220812562, 2.000000000000000000 ) ) ;
#28430=CARTESIAN_POINT ( 'NONE',  ( 0.000000000000000000, 0.000000000000000000, 85.00000000000000000 ) ) ;
#28459=ORIENTED_EDGE ( 'NONE', *, *, #29225, .T. ) ;
#28463=EDGE_CURVE ( 'NONE', #67388, #2651, #48073, .T. ) ;
#28471=DIRECTION ( 'NONE',  ( 0.000000000000000000, -0.000000000000000000, -1.000000000000000000 ) ) ;
#28474=LINE ( 'NONE', #17575, #5725 ) ;
#28480=CARTESIAN_POINT ( 'NONE',  ( -36.11269837220809364, -15.55634918610397754, 85.00100000000000477 ) ) ;
#28507=ORIENTED_EDGE ( 'NONE', *, *, #67432, .T. ) ;
#28541=LINE ( 'NONE', #66542, #28890 ) ;
#28550=DIRECTION ( 'NONE',  ( 0.000000000000000000, -1.000000000000000000, 0.000000000000000000 ) ) ;
#28556=VECTOR ( 'NONE', #7458, 1000.000000000000000 ) ;
#28578=ORIENTED_EDGE ( 'NONE', *, *, #50654, .F. ) ;
#28589=ORIENTED_EDGE ( 'NONE', *, *, #19182, .F. ) ;
#28604=EDGE_CURVE ( 'NONE', #15890, #10200, #45588, .T. ) ;
#28605=PLANE ( 'NONE',  #166 ) ;
#28610=ORIENTED_EDGE ( 'NONE', *, *, #5690, .F. ) ;
#28663=ORIENTED_EDGE ( 'NONE', *, *, #632, .F. ) ;
#28666=EDGE_CURVE ( 'NONE', #51932, #5346, #60723, .T. ) ;
#28688=VECTOR ( 'NONE', #26443, 1000.000000000000000 ) ;
#28693=ADVANCED_FACE ( 'NONE', ( #41358 ), #10031, .F. ) ;
#28709=EDGE_LOOP ( 'NONE', ( #1351, #21069, #7850, #22419 ) ) ;
#28718=CARTESIAN_POINT ( 'NONE',  ( -31.11269837220804035, 15.55634918610408945, 2.000000000000001776 ) ) ;
#28730=ADVANCED_FACE ( 'NONE', ( #35739 ), #47299, .F. ) ;
#28742=DIRECTION ( 'NONE',  ( -0.000000000000000000, -1.000000000000000000, -0.000000000000000000 ) ) ;
#28748=VECTOR ( 'NONE', #5104, 1000.000000000000000 ) ;
#28764=EDGE_CURVE ( 'NONE', #40747, #67789, #38401, .T. ) ;
#28780=FACE_BOUND ( 'NONE', #49994, .T. ) ;
#28789=AXIS2_PLACEMENT_3D ( 'NONE', #33737, #56572, #13661 ) ;
#28817=PLANE ( 'NONE',  #3805 ) ;
#28822=ORIENTED_EDGE ( 'NONE', *, *, #4611, .T. ) ;
#28859=VERTEX_POINT ( 'NONE', #34542 ) ;
#28862=EDGE_CURVE ( 'NONE', #19609, #13387, #62292, .T. ) ;
#28883=CARTESIAN_POINT ( 'NONE',  ( 0.000000000000000000, 0.000000000000000000, -0.002000000000002000178 ) ) ;
#28888=LINE ( 'NONE', #50340, #29788 ) ;
#28890=VECTOR ( 'NONE', #45409, 1000.000000000000000 ) ;
#28893=CARTESIAN_POINT ( 'NONE',  ( -31.11269837220804035, 15.55634918610408945, 85.00100000000000477 ) ) ;
#28896=CARTESIAN_POINT ( 'NONE',  ( -15.55634918610403439, 5.000000000000028422, 85.00100000000000477 ) ) ;
#28903=VECTOR ( 'NONE', #15480, 1000.000000000000000 ) ;
#28912=EDGE_CURVE ( 'NONE', #58260, #16366, #25016, .T. ) ;
#28934=CARTESIAN_POINT ( 'NONE',  ( 26.11269837220806167, 4.999999999999936939, 0.000000000000000000 ) ) ;
#28939=ORIENTED_EDGE ( 'NONE', *, *, #31868, .T. ) ;
#28941=LINE ( 'NONE', #29616, #10640 ) ;
#28960=DIRECTION ( 'NONE',  ( 0.000000000000000000, -0.000000000000000000, -1.000000000000000000 ) ) ;
#28964=ORIENTED_EDGE ( 'NONE', *, *, #9200, .F. ) ;
#28965=EDGE_LOOP ( 'NONE', ( #38705, #1653, #22607, #30150 ) ) ;
#29017=ORIENTED_EDGE ( 'NONE', *, *, #48965, .F. ) ;
#29021=PLANE ( 'NONE',  #46712 ) ;
#29024=ORIENTED_EDGE ( 'NONE', *, *, #49589, .F. ) ;
#29029=LINE ( 'NONE', #44126, #18460 ) ;
#29055=DIRECTION ( 'NONE',  ( -0.000000000000000000, -0.000000000000000000, -1.000000000000000000 ) ) ;
#29092=EDGE_CURVE ( 'NONE', #46344, #32718, #57709, .T. ) ;
#29110=DIRECTION ( 'NONE',  ( 0.000000000000000000, -1.000000000000000000, 0.000000000000000000 ) ) ;
#29122=ORIENTED_EDGE ( 'NONE', *, *, #42561, .F. ) ;
#29132=EDGE_LOOP ( 'NONE', ( #60808, #35010, #19871, #49410 ) ) ;
#29160=CARTESIAN_POINT ( 'NONE',  ( -31.11269837220804035, 20.55634918610408945, 85.00100000000000477 ) ) ;
#29176=ORIENTED_EDGE ( 'NONE', *, *, #23911, .F. ) ;
#29192=VECTOR ( 'NONE', #17138, 999.9999999999998863 ) ;
#29193=ORIENTED_EDGE ( 'NONE', *, *, #22283, .F. ) ;
#29225=EDGE_CURVE ( 'NONE', #10970, #19049, #15062, .T. ) ;
#29248=DIRECTION ( 'NONE',  ( 0.000000000000000000, 1.000000000000000000, -0.000000000000000000 ) ) ;
#29255=EDGE_CURVE ( 'NONE', #39331, #33627, #15407, .T. ) ;
#29276=ORIENTED_EDGE ( 'NONE', *, *, #48469, .T. ) ;
#29341=EDGE_CURVE ( 'NONE', #11433, #34620, #26986, .T. ) ;
#29346=VECTOR ( 'NONE', #33594, 1000.000000000000000 ) ;
#29361=FACE_OUTER_BOUND ( 'NONE', #23913, .T. ) ;
#29379=PLANE ( 'NONE',  #15239 ) ;
#29402=CARTESIAN_POINT ( 'NONE',  ( 15.55634918610400241, -15.55634918610406103, 0.000000000000000000 ) ) ;
#29438=FACE_OUTER_BOUND ( 'NONE', #36588, .T. ) ;
#29446=CARTESIAN_POINT ( 'NONE',  ( -20.55634918610408945, -31.11269837220804035, 2.000000000000001776 ) ) ;
#29447=VERTEX_POINT ( 'NONE', #22061 ) ;
#29452=ORIENTED_EDGE ( 'NONE', *, *, #16682, .F. ) ;
#29472=ORIENTED_EDGE ( 'NONE', *, *, #33602, .F. ) ;
#29482=VERTEX_POINT ( 'NONE', #13938 ) ;
#29511=ORIENTED_EDGE ( 'NONE', *, *, #62373, .F. ) ;
#29512=CARTESIAN_POINT ( 'NONE',  ( 26.11269837220809364, 15.55634918610396866, 85.00100000000000477 ) ) ;
#29591=VECTOR ( 'NONE', #37881, 1000.000000000000000 ) ;
#29592=LINE ( 'NONE', #2871, #17215 ) ;
#29616=CARTESIAN_POINT ( 'NONE',  ( 46.66904755831207297, -10.55634918610412853, 0.000000000000000000 ) ) ;
#29630=FACE_OUTER_BOUND ( 'NONE', #60747, .T. ) ;
#29634=ORIENTED_EDGE ( 'NONE', *, *, #23112, .T. ) ;
#29637=EDGE_CURVE ( 'NONE', #45426, #7527, #8051, .T. ) ;
#29656=CARTESIAN_POINT ( 'NONE',  ( 10.55634918610397577, -26.11269837220809364, 0.000000000000000000 ) ) ;
#29666=CARTESIAN_POINT ( 'NONE',  ( -36.11269837220801548, 36.11269837220812207, 2.000000000000001776 ) ) ;
#29687=ADVANCED_FACE ( 'NONE', ( #7717 ), #61521, .F. ) ;
#29693=LINE ( 'NONE', #35674, #53175 ) ;
#29694=DIRECTION ( 'NONE',  ( 1.000000000000000000, 0.000000000000000000, 0.000000000000000000 ) ) ;
#29752=CIRCLE ( 'NONE', #8422, 66.50000000000000000 ) ;
#29781=ORIENTED_EDGE ( 'NONE', *, *, #66157, .T. ) ;
#29788=VECTOR ( 'NONE', #34169, 1000.000000000000000 ) ;
#29798=VECTOR ( 'NONE', #23458, 1000.000000000000000 ) ;
#29801=CARTESIAN_POINT ( 'NONE',  ( 72.99999999999998579, 8.939921633775675282E-15, 25.70156211871649887 ) ) ;
#29805=VECTOR ( 'NONE', #21649, 1000.000000000000000 ) ;
#29823=DIRECTION ( 'NONE',  ( -0.000000000000000000, -0.000000000000000000, -1.000000000000000000 ) ) ;
#29825=DIRECTION ( 'NONE',  ( 0.000000000000000000, 0.000000000000000000, -1.000000000000000000 ) ) ;
#29828=CARTESIAN_POINT ( 'NONE',  ( -4.999999999999922728, 46.66904755831208718, 85.00100000000000477 ) ) ;
#29896=VECTOR ( 'NONE', #6432, 1000.000000000000000 ) ;
#29903=VECTOR ( 'NONE', #34535, 1000.000000000000000 ) ;
#29904=DIRECTION ( 'NONE',  ( -0.000000000000000000, -1.000000000000000000, -0.000000000000000000 ) ) ;
#29923=FACE_OUTER_BOUND ( 'NONE', #11375, .T. ) ;
#29924=EDGE_LOOP ( 'NONE', ( #22833, #19061, #9550, #56172 ) ) ;
#29955=ADVANCED_FACE ( 'NONE', ( #63934 ), #41452, .F. ) ;
#29957=ORIENTED_EDGE ( 'NONE', *, *, #68405, .F. ) ;
#29966=EDGE_LOOP ( 'NONE', ( #19144, #16859, #38336, #51346 ) ) ;
#29999=AXIS2_PLACEMENT_3D ( 'NONE', #34090, #8039, #34449 ) ;
#30007=ORIENTED_EDGE ( 'NONE', *, *, #53757, .F. ) ;
#30024=DIRECTION ( 'NONE',  ( 0.000000000000000000, 0.000000000000000000, 1.000000000000000000 ) ) ;
#30050=EDGE_CURVE ( 'NONE', #41880, #1454, #32616, .T. ) ;
#30054=EDGE_CURVE ( 'NONE', #3625, #58133, #59237, .T. ) ;
#30067=CARTESIAN_POINT ( 'NONE',  ( -31.11269837220806878, 5.594483210025202879E-14, 85.00100000000000477 ) ) ;
#30075=CARTESIAN_POINT ( 'NONE',  ( 31.11269837220800127, -31.11269837220812562, 0.000000000000000000 ) ) ;
#30076=CARTESIAN_POINT ( 'NONE',  ( 0.000000000000000000, 0.000000000000000000, 85.00000000000000000 ) ) ;
#30088=CARTESIAN_POINT ( 'NONE',  ( -20.55634918610411077, -46.66904755831208718, 85.00100000000000477 ) ) ;
#30095=VERTEX_POINT ( 'NONE', #11151 ) ;
#30103=CARTESIAN_POINT ( 'NONE',  ( 15.55634918610409656, 36.11269837220803680, 85.00100000000000477 ) ) ;
#30112=AXIS2_PLACEMENT_3D ( 'NONE', #46504, #41246, #62703 ) ;
#30136=ADVANCED_FACE ( 'NONE', ( #67670 ), #63071, .F. ) ;
#30150=ORIENTED_EDGE ( 'NONE', *, *, #26122, .F. ) ;
#30196=CONICAL_SURFACE ( 'NONE', #40281, 74.99999999999998579, 0.6747409422235518539 ) ;
#30210=VERTEX_POINT ( 'NONE', #53535 ) ;
#30219=CARTESIAN_POINT ( 'NONE',  ( -15.55634918610400597, 15.55634918610405748, 2.000000000000001776 ) ) ;
#30237=VERTEX_POINT ( 'NONE', #26130 ) ;
#30242=EDGE_LOOP ( 'NONE', ( #14308, #1916, #43778, #40502 ) ) ;
#30252=PLANE ( 'NONE',  #12976 ) ;
#30303=DIRECTION ( 'NONE',  ( -0.000000000000000000, -0.000000000000000000, -1.000000000000000000 ) ) ;
#30322=ORIENTED_EDGE ( 'NONE', *, *, #12242, .F. ) ;
#30345=CARTESIAN_POINT ( 'NONE',  ( 10.55634918610396511, -41.66904755831214402, 2.000000000000001776 ) ) ;
#30348=DIRECTION ( 'NONE',  ( 0.000000000000000000, 1.000000000000000000, -0.000000000000000000 ) ) ;
#30391=ORIENTED_EDGE ( 'NONE', *, *, #2926, .F. ) ;
#30398=CARTESIAN_POINT ( 'NONE',  ( -4.999999999999922728, 46.66904755831208718, 0.000000000000000000 ) ) ;
#30412=DIRECTION ( 'NONE',  ( 0.000000000000000000, -0.000000000000000000, -1.000000000000000000 ) ) ;
#30419=VERTEX_POINT ( 'NONE', #46810 ) ;
#30429=CARTESIAN_POINT ( 'NONE',  ( 46.66904755831207297, -10.55634918610412853, 2.000000000000001776 ) ) ;
#30446=ORIENTED_EDGE ( 'NONE', *, *, #67432, .F. ) ;
#30451=LINE ( 'NONE', #61258, #50277 ) ;
#30459=DIRECTION ( 'NONE',  ( 0.000000000000000000, 0.000000000000000000, 1.000000000000000000 ) ) ;
#30475=EDGE_CURVE ( 'NONE', #58133, #3625, #45761, .T. ) ;
#30502=DIRECTION ( 'NONE',  ( 0.000000000000000000, 0.000000000000000000, 1.000000000000000000 ) ) ;
#30503=EDGE_LOOP ( 'NONE', ( #11628, #5798, #59529, #57656 ) ) ;
#30517=DIRECTION ( 'NONE',  ( 0.000000000000000000, 1.000000000000000000, -0.000000000000000000 ) ) ;
#30541=CARTESIAN_POINT ( 'NONE',  ( -15.55634918610403439, 5.000000000000028422, 2.000000000000001776 ) ) ;
#30570=AXIS2_PLACEMENT_3D ( 'NONE', #1420, #22878, #43621 ) ;
#30585=EDGE_CURVE ( 'NONE', #18908, #28859, #12649, .T. ) ;
#30624=FACE_OUTER_BOUND ( 'NONE', #49099, .T. ) ;
#30631=VERTEX_POINT ( 'NONE', #50283 ) ;
#30645=ADVANCED_FACE ( 'NONE', ( #23555 ), #16863, .F. ) ;
#30657=VERTEX_POINT ( 'NONE', #1047 ) ;
#30660=ORIENTED_EDGE ( 'NONE', *, *, #33696, .T. ) ;
#30666=EDGE_LOOP ( 'NONE', ( #41401, #62306, #20182, #66419 ) ) ;
#30677=PLANE ( 'NONE',  #51627 ) ;
#30692=DIRECTION ( 'NONE',  ( 0.000000000000000000, 1.000000000000000000, -0.000000000000000000 ) ) ;
#30715=VECTOR ( 'NONE', #28383, 1000.000000000000000 ) ;
#30721=DIRECTION ( 'NONE',  ( 0.000000000000000000, 0.000000000000000000, 1.000000000000000000 ) ) ;
#30727=LINE ( 'NONE', #25801, #41901 ) ;
#30734=ORIENTED_EDGE ( 'NONE', *, *, #60272, .F. ) ;
#30735=CARTESIAN_POINT ( 'NONE',  ( -31.11269837220812207, -26.11269837220801193, 85.00100000000000477 ) ) ;
#30769=DIRECTION ( 'NONE',  ( 0.000000000000000000, -0.000000000000000000, -1.000000000000000000 ) ) ;
#30770=ORIENTED_EDGE ( 'NONE', *, *, #1915, .T. ) ;
#30795=VERTEX_POINT ( 'NONE', #2789 ) ;
#30808=VERTEX_POINT ( 'NONE', #56951 ) ;
#30810=PLANE ( 'NONE',  #19488 ) ;
#30831=DIRECTION ( 'NONE',  ( 0.000000000000000000, 1.000000000000000000, -0.000000000000000000 ) ) ;
#30846=ORIENTED_EDGE ( 'NONE', *, *, #11689, .F. ) ;
#30855=DIRECTION ( 'NONE',  ( 1.000000000000000000, 0.000000000000000000, -0.000000000000000000 ) ) ;
#30881=ADVANCED_FACE ( 'NONE', ( #31259 ), #25975, .F. ) ;
#30890=VERTEX_POINT ( 'NONE', #44205 ) ;
#30921=EDGE_CURVE ( 'NONE', #48044, #17255, #11495, .T. ) ;
#30936=DIRECTION ( 'NONE',  ( -1.000000000000000000, 0.000000000000000000, 0.000000000000000000 ) ) ;
#30954=DIRECTION ( 'NONE',  ( 0.000000000000000000, 0.000000000000000000, 1.000000000000000000 ) ) ;
#30956=AXIS2_PLACEMENT_3D ( 'NONE', #19031, #23965, #66899 ) ;
#30977=CARTESIAN_POINT ( 'NONE',  ( -7.329206686002009974E-14, -41.66904755831212270, 85.00100000000000477 ) ) ;
#31019=AXIS2_PLACEMENT_3D ( 'NONE', #8469, #51381, #3196 ) ;
#31029=CARTESIAN_POINT ( 'NONE',  ( -4.999999999999922728, 51.66904755831208718, 85.00100000000000477 ) ) ;
#31055=VECTOR ( 'NONE', #67069, 1000.000000000000000 ) ;
#31059=VECTOR ( 'NONE', #35842, 1000.000000000000000 ) ;
#31074=ADVANCED_FACE ( 'NONE', ( #61446 ), #67770, .F. ) ;
#31079=FACE_OUTER_BOUND ( 'NONE', #46396, .T. ) ;
#31091=DIRECTION ( 'NONE',  ( 0.000000000000000000, 1.000000000000000000, -0.000000000000000000 ) ) ;
#31102=DIRECTION ( 'NONE',  ( 0.000000000000000000, 1.000000000000000000, -0.000000000000000000 ) ) ;
#31110=LINE ( 'NONE', #42679, #6897 ) ;
#31113=ORIENTED_EDGE ( 'NONE', *, *, #52807, .F. ) ;
#31126=EDGE_LOOP ( 'NONE', ( #52310, #37276, #30446, #15278 ) ) ;
#31132=DIRECTION ( 'NONE',  ( 0.000000000000000000, 1.000000000000000000, -0.000000000000000000 ) ) ;
#31174=ORIENTED_EDGE ( 'NONE', *, *, #52390, .T. ) ;
#31195=DIRECTION ( 'NONE',  ( 0.000000000000000000, 0.000000000000000000, 1.000000000000000000 ) ) ;
#31198=VECTOR ( 'NONE', #28191, 1000.000000000000000 ) ;
#31206=PLANE ( 'NONE',  #55295 ) ;
#31207=VECTOR ( 'NONE', #42929, 1000.000000000000000 ) ;
#31218=EDGE_CURVE ( 'NONE', #35061, #17896, #38507, .T. ) ;
#31219=DIRECTION ( 'NONE',  ( 0.000000000000000000, 0.000000000000000000, 1.000000000000000000 ) ) ;
#31233=LINE ( 'NONE', #56928, #50936 ) ;
#31234=EDGE_CURVE ( 'NONE', #62926, #30795, #59952, .T. ) ;
#31259=FACE_OUTER_BOUND ( 'NONE', #64042, .T. ) ;
#31261=ORIENTED_EDGE ( 'NONE', *, *, #33936, .T. ) ;
#31289=ADVANCED_FACE ( 'NONE', ( #61701 ), #66317, .F. ) ;
#31298=VECTOR ( 'NONE', #6326, 1000.000000000000000 ) ;
#31305=DIRECTION ( 'NONE',  ( -0.000000000000000000, -0.000000000000000000, -1.000000000000000000 ) ) ;
#31310=ORIENTED_EDGE ( 'NONE', *, *, #5761, .F. ) ;
#31326=EDGE_LOOP ( 'NONE', ( #6665, #26349, #67446, #6952 ) ) ;
#31359=EDGE_LOOP ( 'NONE', ( #54915, #41905, #11024, #69509 ) ) ;
#31377=DIRECTION ( 'NONE',  ( 0.000000000000000000, -1.000000000000000000, 0.000000000000000000 ) ) ;
#31428=EDGE_LOOP ( 'NONE', ( #47181, #21986, #49418, #34237 ) ) ;
#31468=ORIENTED_EDGE ( 'NONE', *, *, #18972, .T. ) ;
#31490=ORIENTED_EDGE ( 'NONE', *, *, #23846, .F. ) ;
#31504=VECTOR ( 'NONE', #18078, 1000.000000000000000 ) ;
#31529=CARTESIAN_POINT ( 'NONE',  ( 6.375108774214766072E-14, 36.11269837220805812, 85.00100000000000477 ) ) ;
#31530=ORIENTED_EDGE ( 'NONE', *, *, #52485, .T. ) ;
#31533=LINE ( 'NONE', #20975, #39232 ) ;
#31548=AXIS2_PLACEMENT_3D ( 'NONE', #8586, #36344, #20163 ) ;
#31580=DIRECTION ( 'NONE',  ( -0.000000000000000000, -0.000000000000000000, -1.000000000000000000 ) ) ;
#31587=EDGE_CURVE ( 'NONE', #35180, #10168, #36357, .T. ) ;
#31591=DIRECTION ( 'NONE',  ( 0.000000000000000000, -1.000000000000000000, 0.000000000000000000 ) ) ;
#31608=VECTOR ( 'NONE', #27109, 1000.000000000000000 ) ;
#31609=AXIS2_PLACEMENT_3D ( 'NONE', #56400, #35990, #46186 ) ;
#31618=( GEOMETRIC_REPRESENTATION_CONTEXT ( 3 ) GLOBAL_UNCERTAINTY_ASSIGNED_CONTEXT ( ( #47224 ) ) GLOBAL_UNIT_ASSIGNED_CONTEXT ( ( #27565, #43733, #22644 ) ) REPRESENTATION_CONTEXT ( 'NONE', 'WORKASPACE' ) );
#31619=CARTESIAN_POINT ( 'NONE',  ( 10.55634918610400419, -10.55634918610406281, 85.00100000000000477 ) ) ;
#31660=VECTOR ( 'NONE', #2660, 1000.000000000000000 ) ;
#31661=PLANE ( 'NONE',  #18837 ) ;
#31678=ORIENTED_EDGE ( 'NONE', *, *, #12801, .F. ) ;
#31680=CARTESIAN_POINT ( 'NONE',  ( 10.55634918610396511, -46.66904755831214402, 85.00100000000000477 ) ) ;
#31692=EDGE_CURVE ( 'NONE', #54421, #61065, #39387, .T. ) ;
#31701=VERTEX_POINT ( 'NONE', #27783 ) ;
#31702=VECTOR ( 'NONE', #6283, 1000.000000000000000 ) ;
#31732=CARTESIAN_POINT ( 'NONE',  ( 46.66904755831212981, 15.55634918610394379, 2.000000000000001776 ) ) ;
#31755=EDGE_CURVE ( 'NONE', #22892, #21953, #49222, .T. ) ;
#31759=AXIS2_PLACEMENT_3D ( 'NONE', #14874, #46189, #30721 ) ;
#31796=ORIENTED_EDGE ( 'NONE', *, *, #55046, .F. ) ;
#31799=VERTEX_POINT ( 'NONE', #61539 ) ;
#31805=VECTOR ( 'NONE', #28742, 1000.000000000000000 ) ;
#31840=CARTESIAN_POINT ( 'NONE',  ( 26.11269837220800127, -26.11269837220812562, 85.00100000000000477 ) ) ;
#31845=ORIENTED_EDGE ( 'NONE', *, *, #62681, .F. ) ;
#31858=AXIS2_PLACEMENT_3D ( 'NONE', #50379, #24348, #14124 ) ;
#31868=EDGE_CURVE ( 'NONE', #16148, #34252, #13695, .T. ) ;
#31877=FACE_BOUND ( 'NONE', #67643, .T. ) ;
#31883=CARTESIAN_POINT ( 'NONE',  ( 26.11269837220809364, 15.55634918610396866, 2.000000000000001776 ) ) ;
#31898=CARTESIAN_POINT ( 'NONE',  ( -20.55634918610405748, -10.55634918610400597, 0.000000000000000000 ) ) ;
#31902=CARTESIAN_POINT ( 'NONE',  ( -15.55634918610408945, -31.11269837220804035, 0.000000000000000000 ) ) ;
#31910=VECTOR ( 'NONE', #22261, 1000.000000000000000 ) ;
#31921=DIRECTION ( 'NONE',  ( -0.000000000000000000, -0.000000000000000000, -1.000000000000000000 ) ) ;
#31948=VECTOR ( 'NONE', #20624, 1000.000000000000000 ) ;
#31952=DIRECTION ( 'NONE',  ( -1.000000000000000000, 0.000000000000000000, 0.000000000000000000 ) ) ;
#31973=LINE ( 'NONE', #42851, #66232 ) ;
#31978=VERTEX_POINT ( 'NONE', #65342 ) ;
#31986=LINE ( 'NONE', #59732, #41811 ) ;
#32007=DIRECTION ( 'NONE',  ( 0.000000000000000000, -0.000000000000000000, -1.000000000000000000 ) ) ;
#32019=EDGE_LOOP ( 'NONE', ( #40217, #5610, #48502, #18083 ) ) ;
#32031=CARTESIAN_POINT ( 'NONE',  ( -31.11269837220804035, 15.55634918610408945, 0.000000000000000000 ) ) ;
#32033=CARTESIAN_POINT ( 'NONE',  ( 7.762887554996211747E-14, 46.66904755831208718, 2.000000000000001776 ) ) ;
#32046=VECTOR ( 'NONE', #37457, 1000.000000000000000 ) ;
#32057=DIRECTION ( 'NONE',  ( 1.000000000000000000, 0.000000000000000000, 0.000000000000000000 ) ) ;
#32062=CARTESIAN_POINT ( 'NONE',  ( -15.55634918610403439, 2.818925648462311528E-14, 85.00100000000000477 ) ) ;
#32073=ORIENTED_EDGE ( 'NONE', *, *, #44284, .F. ) ;
#32076=CARTESIAN_POINT ( 'NONE',  ( -5.000000000000073719, -46.66904755831211560, 85.00100000000000477 ) ) ;
#32082=CARTESIAN_POINT ( 'NONE',  ( 46.66904755831210139, 0.000000000000000000, 0.000000000000000000 ) ) ;
#32109=AXIS2_PLACEMENT_3D ( 'NONE', #7143, #22981, #49338 ) ;
#32112=CARTESIAN_POINT ( 'NONE',  ( 0.000000000000000000, 0.000000000000000000, -0.002000000000002000178 ) ) ;
#32115=DIRECTION ( 'NONE',  ( 1.000000000000000000, 0.000000000000000000, 0.000000000000000000 ) ) ;
#32127=PLANE ( 'NONE',  #62593 ) ;
#32133=ORIENTED_EDGE ( 'NONE', *, *, #10290, .F. ) ;
#32174=ORIENTED_EDGE ( 'NONE', *, *, #3173, .T. ) ;
#32184=ORIENTED_EDGE ( 'NONE', *, *, #39300, .F. ) ;
#32193=CARTESIAN_POINT ( 'NONE',  ( 15.55634918610406103, 15.55634918610400241, 0.000000000000000000 ) ) ;
#32198=CARTESIAN_POINT ( 'NONE',  ( -4.999999999999936939, 31.11269837220806167, 0.000000000000000000 ) ) ;
#32206=CARTESIAN_POINT ( 'NONE',  ( -15.55634918610411077, -46.66904755831208718, 2.000000000000001776 ) ) ;
#32210=EDGE_LOOP ( 'NONE', ( #42061, #17684, #63432, #34788 ) ) ;
#32211=ORIENTED_EDGE ( 'NONE', *, *, #43017, .F. ) ;
#32270=ADVANCED_FACE ( 'NONE', ( #891 ), #30196, .T. ) ;
#32277=EDGE_CURVE ( 'NONE', #27210, #14795, #33953, .T. ) ;
#32305=VECTOR ( 'NONE', #33450, 1000.000000000000000 ) ;
#32327=ORIENTED_EDGE ( 'NONE', *, *, #12726, .T. ) ;
#32344=CARTESIAN_POINT ( 'NONE',  ( -20.55634918610400419, 15.55634918610405748, 85.00100000000000477 ) ) ;
#32347=FACE_OUTER_BOUND ( 'NONE', #24116, .T. ) ;
#32355=ORIENTED_EDGE ( 'NONE', *, *, #54860, .F. ) ;
#32362=LINE ( 'NONE', #58724, #54371 ) ;
#32376=ORIENTED_EDGE ( 'NONE', *, *, #34324, .F. ) ;
#32392=VERTEX_POINT ( 'NONE', #38882 ) ;
#32409=ADVANCED_FACE ( 'NONE', ( #65255 ), #60675, .F. ) ;
#32423=VERTEX_POINT ( 'NONE', #7215 ) ;
#32426=CARTESIAN_POINT ( 'NONE',  ( -54.99999999999995026, 7.960204194457792519E-15, 0.000000000000000000 ) ) ;
#32436=ORIENTED_EDGE ( 'NONE', *, *, #56304, .T. ) ;
#32448=DIRECTION ( 'NONE',  ( -0.000000000000000000, -0.000000000000000000, 1.000000000000000000 ) ) ;
#32453=ORIENTED_EDGE ( 'NONE', *, *, #32554, .T. ) ;
#32457=CARTESIAN_POINT ( 'NONE',  ( -5.000000000000073719, -46.66904755831211560, 2.000000000000001776 ) ) ;
#32482=LINE ( 'NONE', #53914, #111 ) ;
#32484=FACE_BOUND ( 'NONE', #1283, .T. ) ;
#32522=( NAMED_UNIT ( * ) SI_UNIT ( $, .STERADIAN. ) SOLID_ANGLE_UNIT ( ) );
#32523=ADVANCED_FACE ( 'NONE', ( #29361 ), #39914, .F. ) ;
#32546=ORIENTED_EDGE ( 'NONE', *, *, #67973, .T. ) ;
#32554=EDGE_CURVE ( 'NONE', #25366, #66496, #13195, .T. ) ;
#32565=EDGE_CURVE ( 'NONE', #1235, #53714, #45887, .T. ) ;
#32583=VERTEX_POINT ( 'NONE', #40602 ) ;
#32604=CARTESIAN_POINT ( 'NONE',  ( -51.66904755831212981, -15.55634918610397222, 2.000000000000001776 ) ) ;
#32611=EDGE_CURVE ( 'NONE', #23144, #32692, #67016, .T. ) ;
#32616=LINE ( 'NONE', #39887, #41288 ) ;
#32640=LINE ( 'NONE', #47088, #15044 ) ;
#32689=CARTESIAN_POINT ( 'NONE',  ( 0.000000000000000000, 0.000000000000000000, 0.000000000000000000 ) ) ;
#32692=VERTEX_POINT ( 'NONE', #57480 ) ;
#32712=CARTESIAN_POINT ( 'NONE',  ( -31.11269837220812207, -31.11269837220801193, 0.000000000000000000 ) ) ;
#32718=VERTEX_POINT ( 'NONE', #69409 ) ;
#32720=VERTEX_POINT ( 'NONE', #9642 ) ;
#32778=ORIENTED_EDGE ( 'NONE', *, *, #23667, .F. ) ;
#32786=ORIENTED_EDGE ( 'NONE', *, *, #68683, .T. ) ;
#32797=ADVANCED_FACE ( 'NONE', ( #20186 ), #63100, .F. ) ;
#32804=CARTESIAN_POINT ( 'NONE',  ( -20.55634918610400419, 20.55634918610405748, 85.00100000000000477 ) ) ;
#32811=VECTOR ( 'NONE', #38292, 1000.000000000000000 ) ;
#32821=CARTESIAN_POINT ( 'NONE',  ( 31.11269837220800127, -31.11269837220812562, 85.00100000000000477 ) ) ;
#32824=CARTESIAN_POINT ( 'NONE',  ( -4.999999999999971578, 15.55634918610403084, 2.000000000000000000 ) ) ;
#32839=LINE ( 'NONE', #5417, #23078 ) ;
#32845=ORIENTED_EDGE ( 'NONE', *, *, #36922, .F. ) ;
#32847=VECTOR ( 'NONE', #64045, 1000.000000000000000 ) ;
#32869=ORIENTED_EDGE ( 'NONE', *, *, #4701, .F. ) ;
#32871=LINE ( 'NONE', #27586, #7962 ) ;
#32881=CARTESIAN_POINT ( 'NONE',  ( -51.66904755831210139, 0.000000000000000000, 2.000000000000000000 ) ) ;
#32895=ORIENTED_EDGE ( 'NONE', *, *, #32565, .F. ) ;
#32896=LINE ( 'NONE', #53295, #14369 ) ;
#32907=FACE_BOUND ( 'NONE', #22522, .T. ) ;
#32922=CARTESIAN_POINT ( 'NONE',  ( 31.11269837220806522, -6.375108774214766072E-14, 2.000000000000001776 ) ) ;
#32926=ORIENTED_EDGE ( 'NONE', *, *, #6766, .F. ) ;
#32929=DIRECTION ( 'NONE',  ( 1.000000000000000000, -0.000000000000000000, -0.000000000000000000 ) ) ;
#32950=AXIS2_PLACEMENT_3D ( 'NONE', #46013, #9428, #62189 ) ;
#32971=EDGE_CURVE ( 'NONE', #23803, #5602, #18988, .T. ) ;
#32974=EDGE_LOOP ( 'NONE', ( #48410, #17502, #34063, #23660 ) ) ;
#32980=ORIENTED_EDGE ( 'NONE', *, *, #31218, .T. ) ;
#32981=DIRECTION ( 'NONE',  ( -1.000000000000000000, 0.000000000000000000, 0.000000000000000000 ) ) ;
#33012=ORIENTED_EDGE ( 'NONE', *, *, #24708, .T. ) ;
#33083=EDGE_LOOP ( 'NONE', ( #4405, #50747, #18574, #32184 ) ) ;
#33085=PLANE ( 'NONE',  #30570 ) ;
#33086=DIRECTION ( 'NONE',  ( 0.000000000000000000, -1.000000000000000000, 0.000000000000000000 ) ) ;
#33095=LINE ( 'NONE', #54173, #35680 ) ;
#33134=VERTEX_POINT ( 'NONE', #4115 ) ;
#33140=DIRECTION ( 'NONE',  ( -0.000000000000000000, -1.000000000000000000, -0.000000000000000000 ) ) ;
#33161=AXIS2_PLACEMENT_3D ( 'NONE', #46168, #30692, #35631 ) ;
#33165=CARTESIAN_POINT ( 'NONE',  ( 10.55634918610403084, 0.000000000000000000, 2.000000000000000000 ) ) ;
#33180=EDGE_CURVE ( 'NONE', #10664, #41218, #31533, .T. ) ;
#33185=DIRECTION ( 'NONE',  ( -0.000000000000000000, -0.000000000000000000, -1.000000000000000000 ) ) ;
#33189=ORIENTED_EDGE ( 'NONE', *, *, #28030, .F. ) ;
#33194=DIRECTION ( 'NONE',  ( -1.000000000000000000, 0.000000000000000000, 0.000000000000000000 ) ) ;
#33203=CYLINDRICAL_SURFACE ( 'NONE', #34039, 72.99999999999998579 ) ;
#33205=ADVANCED_FACE ( 'NONE', ( #45725, #27274, #33275, #64928, #42760, #26597, #65629, #5139, #16722, #37146, #43105, #195, #27977, #11435, #65268, #59976, #5482, #21312, #58589, #64575, #1250, #22702, #10408, #22010, #31877, #64222, #38181, #69494, #49420, #53305, #48033, #6167, #32907, #16035, #59621, #37487 ), #44142, .T. ) ;
#33214=VECTOR ( 'NONE', #440, 1000.000000000000000 ) ;
#33219=VERTEX_POINT ( 'NONE', #54344 ) ;
#33258=VERTEX_POINT ( 'NONE', #553 ) ;
#33263=VECTOR ( 'NONE', #58905, 1000.000000000000000 ) ;
#33264=VECTOR ( 'NONE', #56607, 1000.000000000000000 ) ;
#33271=ORIENTED_EDGE ( 'NONE', *, *, #62086, .F. ) ;
#33275=FACE_BOUND ( 'NONE', #5491, .T. ) ;
#33287=CARTESIAN_POINT ( 'NONE',  ( -5.000000000000058620, -31.11269837220806878, 0.000000000000000000 ) ) ;
#33297=PLANE ( 'NONE',  #46400 ) ;
#33302=FACE_OUTER_BOUND ( 'NONE', #46489, .T. ) ;
#33315=AXIS2_PLACEMENT_3D ( 'NONE', #62463, #58214, #63497 ) ;
#33319=DIRECTION ( 'NONE',  ( -0.000000000000000000, -0.000000000000000000, -1.000000000000000000 ) ) ;
#33326=DIRECTION ( 'NONE',  ( 0.000000000000000000, 0.000000000000000000, -1.000000000000000000 ) ) ;
#33338=ORIENTED_EDGE ( 'NONE', *, *, #41605, .F. ) ;
#33351=ORIENTED_EDGE ( 'NONE', *, *, #51773, .F. ) ;
#33358=EDGE_CURVE ( 'NONE', #22095, #32423, #66342, .T. ) ;
#33390=CARTESIAN_POINT ( 'NONE',  ( -4.999999999999971578, 15.55634918610403084, 85.00100000000000477 ) ) ;
#33391=DIRECTION ( 'NONE',  ( -0.000000000000000000, -1.000000000000000000, -0.000000000000000000 ) ) ;
#33401=DIRECTION ( 'NONE',  ( 0.000000000000000000, -1.000000000000000000, 0.000000000000000000 ) ) ;
#33413=ORIENTED_EDGE ( 'NONE', *, *, #67973, .F. ) ;
#33421=VECTOR ( 'NONE', #38018, 1000.000000000000000 ) ;
#33430=CARTESIAN_POINT ( 'NONE',  ( 10.55634918610396511, -46.66904755831214402, 2.000000000000000000 ) ) ;
#33431=DIRECTION ( 'NONE',  ( -1.000000000000000000, 0.000000000000000000, 0.000000000000000000 ) ) ;
#33437=DIRECTION ( 'NONE',  ( -1.000000000000000000, 0.000000000000000000, 0.000000000000000000 ) ) ;
#33439=ADVANCED_FACE ( 'NONE', ( #26169 ), #9997, .T. ) ;
#33440=CARTESIAN_POINT ( 'NONE',  ( 10.55634918610403084, 4.999999999999969802, 85.00100000000000477 ) ) ;
#33448=EDGE_LOOP ( 'NONE', ( #13310, #55794, #66940, #1089 ) ) ;
#33450=DIRECTION ( 'NONE',  ( 0.000000000000000000, 1.000000000000000000, 0.000000000000000000 ) ) ;
#33462=CARTESIAN_POINT ( 'NONE',  ( 26.11269837220809364, 15.55634918610396866, 85.00100000000000477 ) ) ;
#33482=PLANE ( 'NONE',  #13825 ) ;
#33497=FACE_OUTER_BOUND ( 'NONE', #24272, .T. ) ;
#33498=CARTESIAN_POINT ( 'NONE',  ( -46.66904755831212981, -10.55634918610397222, 0.000000000000000000 ) ) ;
#33510=EDGE_CURVE ( 'NONE', #39103, #49065, #33662, .T. ) ;
#33527=EDGE_LOOP ( 'NONE', ( #35583, #45930, #54888, #18130 ) ) ;
#33529=LINE ( 'NONE', #56017, #62324 ) ;
#33563=EDGE_LOOP ( 'NONE', ( #69427, #56370, #19780, #21316 ) ) ;
#33567=SURFACE_STYLE_USAGE ( .BOTH. , #17004 ) ;
#33579=DIRECTION ( 'NONE',  ( 0.000000000000000000, -1.000000000000000000, 0.000000000000000000 ) ) ;
#33594=DIRECTION ( 'NONE',  ( 1.000000000000000000, -0.000000000000000000, -0.000000000000000000 ) ) ;
#33602=EDGE_CURVE ( 'NONE', #46713, #38519, #48625, .T. ) ;
#33609=DIRECTION ( 'NONE',  ( -0.000000000000000000, -0.000000000000000000, 1.000000000000000000 ) ) ;
#33627=VERTEX_POINT ( 'NONE', #54255 ) ;
#33662=CIRCLE ( 'NONE', #17934, 65.00000000000000000 ) ;
#33671=CARTESIAN_POINT ( 'NONE',  ( 0.000000000000000000, 0.000000000000000000, 0.000000000000000000 ) ) ;
#33672=LINE ( 'NONE', #20245, #63439 ) ;
#33681=VECTOR ( 'NONE', #37313, 1000.000000000000000 ) ;
#33682=LINE ( 'NONE', #2020, #40791 ) ;
#33686=VERTEX_POINT ( 'NONE', #4295 ) ;
#33691=ADVANCED_FACE ( 'NONE', ( #29630 ), #30677, .F. ) ;
#33696=EDGE_CURVE ( 'NONE', #10168, #53714, #35951, .T. ) ;
#33713=EDGE_LOOP ( 'NONE', ( #58397, #2500 ) ) ;
#33723=FACE_OUTER_BOUND ( 'NONE', #63549, .T. ) ;
#33737=CARTESIAN_POINT ( 'NONE',  ( 6.375108774214766072E-14, 31.11269837220806167, 85.00100000000000477 ) ) ;
#33766=DIRECTION ( 'NONE',  ( 1.000000000000000000, 0.000000000000000000, 0.000000000000000000 ) ) ;
#33796=PLANE ( 'NONE',  #2847 ) ;
#33797=PLANE ( 'NONE',  #66981 ) ;
#33806=DIRECTION ( 'NONE',  ( 0.000000000000000000, 0.000000000000000000, 1.000000000000000000 ) ) ;
#33819=CARTESIAN_POINT ( 'NONE',  ( -15.55634918610403439, 2.818925648462311528E-14, 2.000000000000001776 ) ) ;
#33837=CARTESIAN_POINT ( 'NONE',  ( -15.55634918610403439, 2.818925648462311528E-14, 0.000000000000000000 ) ) ;
#33850=DIRECTION ( 'NONE',  ( 0.000000000000000000, 1.000000000000000000, 0.000000000000000000 ) ) ;
#33853=ADVANCED_FACE ( 'NONE', ( #46493, #19420 ), #2908, .T. ) ;
#33884=PLANE ( 'NONE',  #16333 ) ;
#33893=LINE ( 'NONE', #9924, #22040 ) ;
#33899=ORIENTED_EDGE ( 'NONE', *, *, #24503, .T. ) ;
#33900=CARTESIAN_POINT ( 'NONE',  ( 26.11269837220806167, -6.375108774214766072E-14, 2.000000000000001776 ) ) ;
#33922=EDGE_CURVE ( 'NONE', #48751, #11163, #4968, .T. ) ;
#33936=EDGE_CURVE ( 'NONE', #34238, #61056, #68977, .T. ) ;
#33945=DIRECTION ( 'NONE',  ( 0.000000000000000000, 1.000000000000000000, 0.000000000000000000 ) ) ;
#33953=LINE ( 'NONE', #44495, #11089 ) ;
#33972=DIRECTION ( 'NONE',  ( -1.000000000000000000, 0.000000000000000000, 0.000000000000000000 ) ) ;
#33982=ORIENTED_EDGE ( 'NONE', *, *, #28376, .F. ) ;
#33994=DIRECTION ( 'NONE',  ( 0.000000000000000000, 0.000000000000000000, -1.000000000000000000 ) ) ;
#34010=ORIENTED_EDGE ( 'NONE', *, *, #36472, .F. ) ;
#34014=DIRECTION ( 'NONE',  ( 1.000000000000000000, -0.000000000000000000, -0.000000000000000000 ) ) ;
#34017=ORIENTED_EDGE ( 'NONE', *, *, #54356, .F. ) ;
#34025=ORIENTED_EDGE ( 'NONE', *, *, #62001, .F. ) ;
#34039=AXIS2_PLACEMENT_3D ( 'NONE', #841, #7162, #59910 ) ;
#34041=CARTESIAN_POINT ( 'NONE',  ( 10.55634918610409656, 31.11269837220803325, 0.000000000000000000 ) ) ;
#34052=FACE_BOUND ( 'NONE', #36444, .T. ) ;
#34059=CIRCLE ( 'NONE', #19593, 54.99999999999995026 ) ;
#34063=ORIENTED_EDGE ( 'NONE', *, *, #56296, .F. ) ;
#34079=VECTOR ( 'NONE', #58998, 1000.000000000000000 ) ;
#34084=DIRECTION ( 'NONE',  ( 0.000000000000000000, 0.000000000000000000, 1.000000000000000000 ) ) ;
#34090=CARTESIAN_POINT ( 'NONE',  ( 0.000000000000000000, 0.000000000000000000, 25.00000000000007816 ) ) ;
#34119=CARTESIAN_POINT ( 'NONE',  ( -36.11269837220804391, 20.55634918610408945, 85.00100000000000477 ) ) ;
#34169=DIRECTION ( 'NONE',  ( 0.000000000000000000, 1.000000000000000000, 0.000000000000000000 ) ) ;
#34175=EDGE_CURVE ( 'NONE', #3914, #18610, #31973, .T. ) ;
#34177=LINE ( 'NONE', #28896, #20365 ) ;
#34213=ORIENTED_EDGE ( 'NONE', *, *, #44792, .F. ) ;
#34233=LINE ( 'NONE', #12075, #13879 ) ;
#34237=ORIENTED_EDGE ( 'NONE', *, *, #4740, .F. ) ;
#34238=VERTEX_POINT ( 'NONE', #15108 ) ;
#34252=VERTEX_POINT ( 'NONE', #11192 ) ;
#34296=DIRECTION ( 'NONE',  ( 0.000000000000000000, 0.000000000000000000, -1.000000000000000000 ) ) ;
#34307=DIRECTION ( 'NONE',  ( 1.000000000000000000, 0.000000000000000000, 0.000000000000000000 ) ) ;
#34324=EDGE_CURVE ( 'NONE', #7572, #56265, #35880, .T. ) ;
#34332=VECTOR ( 'NONE', #10077, 1000.000000000000000 ) ;
#34333=FACE_OUTER_BOUND ( 'NONE', #29924, .T. ) ;
#34384=VECTOR ( 'NONE', #34014, 1000.000000000000000 ) ;
#34400=EDGE_LOOP ( 'NONE', ( #57429, #11520, #69271, #48123 ) ) ;
#34427=CARTESIAN_POINT ( 'NONE',  ( -15.55634918610403439, 2.818925648462311528E-14, 85.00100000000000477 ) ) ;
#34442=ORIENTED_EDGE ( 'NONE', *, *, #37088, .F. ) ;
#34449=DIRECTION ( 'NONE',  ( 1.000000000000000000, 0.000000000000000000, 0.000000000000000000 ) ) ;
#34456=LINE ( 'NONE', #29160, #522 ) ;
#34479=FACE_BOUND ( 'NONE', #61649, .T. ) ;
#34534=CONICAL_SURFACE ( 'NONE', #43474, 73.43826238111391547, 0.6747409422235518539 ) ;
#34535=DIRECTION ( 'NONE',  ( 1.000000000000000000, -0.000000000000000000, 0.000000000000000000 ) ) ;
#34541=LINE ( 'NONE', #19375, #50025 ) ;
#34542=CARTESIAN_POINT ( 'NONE',  ( 15.55634918610403261, 4.999999999999969802, 0.000000000000000000 ) ) ;
#34543=DIRECTION ( 'NONE',  ( -0.000000000000000000, -0.000000000000000000, -1.000000000000000000 ) ) ;
#34552=LINE ( 'NONE', #55282, #52919 ) ;
#34554=DIRECTION ( 'NONE',  ( 1.000000000000000000, 0.000000000000000000, 0.000000000000000000 ) ) ;
#34559=ADVANCED_FACE ( 'NONE', ( #16050 ), #68815, .T. ) ;
#34579=EDGE_LOOP ( 'NONE', ( #22086, #8798, #43925, #47959 ) ) ;
#34587=ORIENTED_EDGE ( 'NONE', *, *, #62001, .T. ) ;
#34590=AXIS2_PLACEMENT_3D ( 'NONE', #61991, #52811, #14163 ) ;
#34612=VERTEX_POINT ( 'NONE', #32922 ) ;
#34620=VERTEX_POINT ( 'NONE', #22023 ) ;
#34644=ADVANCED_FACE ( 'NONE', ( #24384 ), #66608, .F. ) ;
#34659=CARTESIAN_POINT ( 'NONE',  ( -15.55634918610396866, 31.11269837220809009, 2.000000000000001776 ) ) ;
#34675=FACE_OUTER_BOUND ( 'NONE', #31428, .T. ) ;
#34676=ORIENTED_EDGE ( 'NONE', *, *, #613, .T. ) ;
#34679=ORIENTED_EDGE ( 'NONE', *, *, #14219, .F. ) ;
#34683=LINE ( 'NONE', #62441, #45167 ) ;
#34690=LINE ( 'NONE', #23776, #5743 ) ;
#34697=DIRECTION ( 'NONE',  ( 0.000000000000000000, -1.000000000000000000, 0.000000000000000000 ) ) ;
#34704=CARTESIAN_POINT ( 'NONE',  ( -5.000000000000000000, 5.000000000000000000, 85.00100000000000477 ) ) ;
#34731=CARTESIAN_POINT ( 'NONE',  ( -36.11269837220812207, -31.11269837220801193, 2.000000000000001776 ) ) ;
#34738=CARTESIAN_POINT ( 'NONE',  ( -72.99999999999998579, 0.000000000000000000, 85.00000000000000000 ) ) ;
#34754=AXIS2_PLACEMENT_3D ( 'NONE', #43120, #63899, #16051 ) ;
#34755=FACE_BOUND ( 'NONE', #62358, .T. ) ;
#34772=CARTESIAN_POINT ( 'NONE',  ( -15.55634918610408945, -31.11269837220804035, 0.000000000000000000 ) ) ;
#34788=ORIENTED_EDGE ( 'NONE', *, *, #1349, .F. ) ;
#34813=DIRECTION ( 'NONE',  ( -1.000000000000000000, 0.000000000000000000, 0.000000000000000000 ) ) ;
#34820=LINE ( 'NONE', #56257, #33264 ) ;
#34829=CARTESIAN_POINT ( 'NONE',  ( 65.00000000000000000, 0.000000000000000000, 15.70156211871650775 ) ) ;
#34830=EDGE_LOOP ( 'NONE', ( #2726, #19893, #11416, #11316 ) ) ;
#34836=AXIS2_PLACEMENT_3D ( 'NONE', #58267, #10085, #10770 ) ;
#34840=ORIENTED_EDGE ( 'NONE', *, *, #64498, .F. ) ;
#34846=CARTESIAN_POINT ( 'NONE',  ( 0.000000000000000000, 0.000000000000000000, 85.00100000000000477 ) ) ;
#34850=CARTESIAN_POINT ( 'NONE',  ( -31.11269837220804035, 20.55634918610408945, 0.000000000000000000 ) ) ;
#34863=ADVANCED_FACE ( 'NONE', ( #6007 ), #37679, .F. ) ;
#34882=LINE ( 'NONE', #2864, #8316 ) ;
#34891=DIRECTION ( 'NONE',  ( -0.000000000000000000, -0.000000000000000000, -1.000000000000000000 ) ) ;
#34893=EDGE_LOOP ( 'NONE', ( #54601, #15487, #2088, #30322 ) ) ;
#34897=FACE_OUTER_BOUND ( 'NONE', #60291, .T. ) ;
#34898=CARTESIAN_POINT ( 'NONE',  ( -2.645453300864630819E-14, -10.55634918610403439, 2.000000000000001776 ) ) ;
#34904=ADVANCED_FACE ( 'NONE', ( #44707 ), #12698, .T. ) ;
#34909=ORIENTED_EDGE ( 'NONE', *, *, #30050, .F. ) ;
#34927=VECTOR ( 'NONE', #24419, 1000.000000000000000 ) ;
#34952=LINE ( 'NONE', #14864, #67438 ) ;
#34985=EDGE_LOOP ( 'NONE', ( #46586, #31261, #7264, #62934 ) ) ;
#34986=VECTOR ( 'NONE', #48544, 1000.000000000000000 ) ;
#35010=ORIENTED_EDGE ( 'NONE', *, *, #59382, .F. ) ;
#35013=DIRECTION ( 'NONE',  ( 1.000000000000000000, -0.000000000000000000, 0.000000000000000000 ) ) ;
#35031=LINE ( 'NONE', #19538, #18360 ) ;
#35040=DIRECTION ( 'NONE',  ( 0.000000000000000000, 0.000000000000000000, 1.000000000000000000 ) ) ;
#35049=ORIENTED_EDGE ( 'NONE', *, *, #28369, .F. ) ;
#35061=VERTEX_POINT ( 'NONE', #51717 ) ;
#35087=FACE_BOUND ( 'NONE', #29132, .T. ) ;
#35107=VERTEX_POINT ( 'NONE', #68583 ) ;
#35161=ORIENTED_EDGE ( 'NONE', *, *, #52093, .T. ) ;
#35170=VECTOR ( 'NONE', #58310, 1000.000000000000000 ) ;
#35174=CARTESIAN_POINT ( 'NONE',  ( -31.11269837220801193, 31.11269837220812207, 0.000000000000000000 ) ) ;
#35180=VERTEX_POINT ( 'NONE', #20737 ) ;
#35184=VECTOR ( 'NONE', #5848, 1000.000000000000000 ) ;
#35206=EDGE_CURVE ( 'NONE', #66816, #19283, #48244, .T. ) ;
#35229=ORIENTED_EDGE ( 'NONE', *, *, #36903, .T. ) ;
#35246=DIRECTION ( 'NONE',  ( -0.000000000000000000, -0.000000000000000000, -1.000000000000000000 ) ) ;
#35251=DIRECTION ( 'NONE',  ( 1.000000000000000000, 0.000000000000000000, 0.000000000000000000 ) ) ;
#35265=ORIENTED_EDGE ( 'NONE', *, *, #64555, .T. ) ;
#35285=LINE ( 'NONE', #23443, #63240 ) ;
#35314=VECTOR ( 'NONE', #12952, 1000.000000000000000 ) ;
#35323=CARTESIAN_POINT ( 'NONE',  ( 7.762887554996211747E-14, 51.66904755831208718, 2.000000000000001776 ) ) ;
#35362=CARTESIAN_POINT ( 'NONE',  ( 10.55634918610403084, -3.079134169858832593E-14, 85.00100000000000477 ) ) ;
#35368=ORIENTED_EDGE ( 'NONE', *, *, #5567, .T. ) ;
#35375=DIRECTION ( 'NONE',  ( 0.000000000000000000, -0.000000000000000000, -1.000000000000000000 ) ) ;
#35383=AXIS2_PLACEMENT_3D ( 'NONE', #36089, #19203, #20246 ) ;
#35395=CARTESIAN_POINT ( 'NONE',  ( 31.11269837220800127, -26.11269837220812562, 0.000000000000000000 ) ) ;
#35415=ORIENTED_EDGE ( 'NONE', *, *, #49589, .T. ) ;
#35418=AXIS2_PLACEMENT_3D ( 'NONE', #9575, #21491, #57412 ) ;
#35424=CARTESIAN_POINT ( 'NONE',  ( -20.55634918610400419, 15.55634918610405748, 0.000000000000000000 ) ) ;
#35425=CARTESIAN_POINT ( 'NONE',  ( -31.11269837220801193, 31.11269837220812207, 85.00100000000000477 ) ) ;
#35466=DIRECTION ( 'NONE',  ( 0.000000000000000000, 0.000000000000000000, 1.000000000000000000 ) ) ;
#35527=VECTOR ( 'NONE', #54536, 1000.000000000000000 ) ;
#35529=DIRECTION ( 'NONE',  ( 0.000000000000000000, 0.000000000000000000, 1.000000000000000000 ) ) ;
#35535=ORIENTED_EDGE ( 'NONE', *, *, #16192, .T. ) ;
#35542=LINE ( 'NONE', #46083, #69185 ) ;
#35562=EDGE_LOOP ( 'NONE', ( #8788, #37796, #60336, #54133 ) ) ;
#35583=ORIENTED_EDGE ( 'NONE', *, *, #15772, .T. ) ;
#35586=DIRECTION ( 'NONE',  ( 1.000000000000000000, -0.000000000000000000, 0.000000000000000000 ) ) ;
#35631=DIRECTION ( 'NONE',  ( 0.000000000000000000, 0.000000000000000000, 1.000000000000000000 ) ) ;
#35646=EDGE_CURVE ( 'NONE', #33134, #913, #19536, .T. ) ;
#35674=CARTESIAN_POINT ( 'NONE',  ( -15.55634918610396866, 36.11269837220808654, 0.000000000000000000 ) ) ;
#35678=CARTESIAN_POINT ( 'NONE',  ( -15.55634918610400597, 20.55634918610405748, 85.00100000000000477 ) ) ;
#35680=VECTOR ( 'NONE', #16901, 1000.000000000000000 ) ;
#35681=VERTEX_POINT ( 'NONE', #40301 ) ;
#35690=EDGE_LOOP ( 'NONE', ( #40328, #39476, #14452, #61165 ) ) ;
#35691=FACE_OUTER_BOUND ( 'NONE', #31126, .T. ) ;
#35697=EDGE_CURVE ( 'NONE', #18069, #11517, #2670, .T. ) ;
#35700=ADVANCED_FACE ( 'NONE', ( #56475 ), #13913, .F. ) ;
#35710=PLANE ( 'NONE',  #43578 ) ;
#35714=PLANE ( 'NONE',  #38380 ) ;
#35716=VECTOR ( 'NONE', #43936, 1000.000000000000000 ) ;
#35723=CARTESIAN_POINT ( 'NONE',  ( 2.905661822261151883E-14, 15.55634918610403084, 2.000000000000001776 ) ) ;
#35729=CARTESIAN_POINT ( 'NONE',  ( -31.11269837220809364, -10.55634918610397932, 2.000000000000001776 ) ) ;
#35732=ORIENTED_EDGE ( 'NONE', *, *, #51845, .T. ) ;
#35739=FACE_OUTER_BOUND ( 'NONE', #59413, .T. ) ;
#35745=ORIENTED_EDGE ( 'NONE', *, *, #47237, .F. ) ;
#35764=CARTESIAN_POINT ( 'NONE',  ( 0.000000000000000000, 0.000000000000000000, 85.00100000000000477 ) ) ;
#35842=DIRECTION ( 'NONE',  ( -1.000000000000000000, 0.000000000000000000, 0.000000000000000000 ) ) ;
#35858=ORIENTED_EDGE ( 'NONE', *, *, #59531, .T. ) ;
#35880=CIRCLE ( 'NONE', #38122, 72.99999999999998579 ) ;
#35881=LINE ( 'NONE', #63308, #42924 ) ;
#35885=DIRECTION ( 'NONE',  ( 1.000000000000000000, -0.000000000000000000, -0.000000000000000000 ) ) ;
#35898=PLANE ( 'NONE',  #61941 ) ;
#35915=EDGE_CURVE ( 'NONE', #13533, #19369, #66287, .T. ) ;
#35940=CARTESIAN_POINT ( 'NONE',  ( 46.66904755831212981, 20.55634918610394379, 0.000000000000000000 ) ) ;
#35947=ORIENTED_EDGE ( 'NONE', *, *, #28030, .T. ) ;
#35951=LINE ( 'NONE', #31029, #7843 ) ;
#35974=DIRECTION ( 'NONE',  ( 0.000000000000000000, 0.000000000000000000, -1.000000000000000000 ) ) ;
#35990=DIRECTION ( 'NONE',  ( 0.000000000000000000, -1.000000000000000000, 0.000000000000000000 ) ) ;
#36051=EDGE_CURVE ( 'NONE', #56852, #59604, #40914, .T. ) ;
#36059=ORIENTED_EDGE ( 'NONE', *, *, #26208, .F. ) ;
#36060=EDGE_CURVE ( 'NONE', #40134, #32392, #19451, .T. ) ;
#36076=EDGE_CURVE ( 'NONE', #64911, #59267, #3621, .T. ) ;
#36089=CARTESIAN_POINT ( 'NONE',  ( 0.000000000000000000, 0.000000000000000000, -0.002000000000002000178 ) ) ;
#36093=VECTOR ( 'NONE', #17865, 1000.000000000000000 ) ;
#36095=EDGE_LOOP ( 'NONE', ( #63347, #61118, #38179, #5603 ) ) ;
#36105=ORIENTED_EDGE ( 'NONE', *, *, #36304, .F. ) ;
#36106=FACE_OUTER_BOUND ( 'NONE', #46330, .T. ) ;
#36107=CARTESIAN_POINT ( 'NONE',  ( -36.11269837220804391, 15.55634918610408945, 0.000000000000000000 ) ) ;
#36113=CARTESIAN_POINT ( 'NONE',  ( -15.55634918610411077, -41.66904755831209428, 0.000000000000000000 ) ) ;
#36115=CARTESIAN_POINT ( 'NONE',  ( -46.66904755831212981, -15.55634918610397222, 2.000000000000001776 ) ) ;
#36119=ORIENTED_EDGE ( 'NONE', *, *, #18590, .T. ) ;
#36128=FACE_BOUND ( 'NONE', #62899, .T. ) ;
#36145=LINE ( 'NONE', #61821, #25479 ) ;
#36167=CARTESIAN_POINT ( 'NONE',  ( 46.66904755831210139, -9.150666335777657423E-14, 0.000000000000000000 ) ) ;
#36173=CARTESIAN_POINT ( 'NONE',  ( -51.66904755831210139, 6.635317295611287136E-14, 0.000000000000000000 ) ) ;
#36183=EDGE_LOOP ( 'NONE', ( #13349, #50762, #25248, #17867 ) ) ;
#36200=VERTEX_POINT ( 'NONE', #2590 ) ;
#36210=LINE ( 'NONE', #31619, #55260 ) ;
#36211=CARTESIAN_POINT ( 'NONE',  ( 2.905661822261151883E-14, 15.55634918610403084, 0.000000000000000000 ) ) ;
#36214=ADVANCED_FACE ( 'NONE', ( #22128 ), #57440, .F. ) ;
#36235=VECTOR ( 'NONE', #61748, 1000.000000000000000 ) ;
#36242=DIRECTION ( 'NONE',  ( 0.000000000000000000, 1.000000000000000000, 0.000000000000000000 ) ) ;
#36265=ORIENTED_EDGE ( 'NONE', *, *, #26991, .T. ) ;
#36279=EDGE_CURVE ( 'NONE', #60290, #8293, #23105, .T. ) ;
#36285=ORIENTED_EDGE ( 'NONE', *, *, #19380, .F. ) ;
#36304=EDGE_CURVE ( 'NONE', #23177, #12488, #43495, .T. ) ;
#36306=FACE_OUTER_BOUND ( 'NONE', #13891, .T. ) ;
#36343=DIRECTION ( 'NONE',  ( 0.000000000000000000, 0.000000000000000000, 1.000000000000000000 ) ) ;
#36344=DIRECTION ( 'NONE',  ( 0.000000000000000000, 1.000000000000000000, -0.000000000000000000 ) ) ;
#36357=LINE ( 'NONE', #57813, #18896 ) ;
#36358=DIRECTION ( 'NONE',  ( -0.000000000000000000, -0.000000000000000000, -1.000000000000000000 ) ) ;
#36377=AXIS2_PLACEMENT_3D ( 'NONE', #14107, #19035, #25020 ) ;
#36382=CARTESIAN_POINT ( 'NONE',  ( -31.11269837220806878, 5.594483210025202879E-14, 2.000000000000001776 ) ) ;
#36397=LINE ( 'NONE', #15629, #10307 ) ;
#36400=DIRECTION ( 'NONE',  ( -0.000000000000000000, -0.000000000000000000, -1.000000000000000000 ) ) ;
#36404=ORIENTED_EDGE ( 'NONE', *, *, #150, .F. ) ;
#36421=CARTESIAN_POINT ( 'NONE',  ( 15.55634918610406103, 15.55634918610400241, 85.00100000000000477 ) ) ;
#36444=EDGE_LOOP ( 'NONE', ( #49405, #46617, #27235, #4012 ) ) ;
#36472=EDGE_CURVE ( 'NONE', #36947, #1035, #32871, .T. ) ;
#36473=FACE_OUTER_BOUND ( 'NONE', #64438, .T. ) ;
#36500=PLANE ( 'NONE',  #32950 ) ;
#36508=FACE_OUTER_BOUND ( 'NONE', #16647, .T. ) ;
#36534=EDGE_CURVE ( 'NONE', #53581, #52273, #39544, .T. ) ;
#36548=DIRECTION ( 'NONE',  ( -0.000000000000000000, -0.000000000000000000, -1.000000000000000000 ) ) ;
#36551=DIRECTION ( 'NONE',  ( 0.000000000000000000, -1.000000000000000000, 0.000000000000000000 ) ) ;
#36560=VERTEX_POINT ( 'NONE', #9264 ) ;
#36561=ADVANCED_FACE ( 'NONE', ( #31079 ), #62387, .F. ) ;
#36573=VECTOR ( 'NONE', #65041, 1000.000000000000000 ) ;
#36577=VECTOR ( 'NONE', #27166, 1000.000000000000000 ) ;
#36585=SHAPE_REPRESENTATION ( 'back cover', ( #66832 ), #51149 ) ;
#36588=EDGE_LOOP ( 'NONE', ( #52309, #53552, #52739, #9306 ) ) ;
#36613=FACE_OUTER_BOUND ( 'NONE', #34579, .T. ) ;
#36629=VECTOR ( 'NONE', #18032, 1000.000000000000000 ) ;
#36662=DIRECTION ( 'NONE',  ( -0.000000000000000000, -0.000000000000000000, -1.000000000000000000 ) ) ;
#36680=DIRECTION ( 'NONE',  ( -0.000000000000000000, -0.000000000000000000, -1.000000000000000000 ) ) ;
#36691=EDGE_CURVE ( 'NONE', #62726, #12932, #13427, .T. ) ;
#36703=EDGE_CURVE ( 'NONE', #23177, #15890, #34552, .T. ) ;
#36744=FACE_OUTER_BOUND ( 'NONE', #45434, .T. ) ;
#36801=VERTEX_POINT ( 'NONE', #63689 ) ;
#36875=EDGE_CURVE ( 'NONE', #39681, #10970, #61183, .T. ) ;
#36895=DIRECTION ( 'NONE',  ( 0.000000000000000000, -1.000000000000000000, 0.000000000000000000 ) ) ;
#36898=EDGE_LOOP ( 'NONE', ( #28939, #48610, #36105, #68039 ) ) ;
#36903=EDGE_CURVE ( 'NONE', #30795, #30237, #49560, .T. ) ;
#36922=EDGE_CURVE ( 'NONE', #3968, #69309, #28474, .T. ) ;
#36924=FACE_OUTER_BOUND ( 'NONE', #32974, .T. ) ;
#36945=FACE_OUTER_BOUND ( 'NONE', #21857, .T. ) ;
#36947=VERTEX_POINT ( 'NONE', #12652 ) ;
#36948=EDGE_CURVE ( 'NONE', #38815, #2018, #61533, .T. ) ;
#36956=DIRECTION ( 'NONE',  ( -1.000000000000000000, 0.000000000000000000, 0.000000000000000000 ) ) ;
#36965=DIRECTION ( 'NONE',  ( -0.000000000000000000, -0.000000000000000000, -1.000000000000000000 ) ) ;
#37013=CARTESIAN_POINT ( 'NONE',  ( -46.66904755831212981, -15.55634918610397222, 85.00100000000000477 ) ) ;
#37019=LINE ( 'NONE', #31732, #18263 ) ;
#37029=FACE_OUTER_BOUND ( 'NONE', #53468, .T. ) ;
#37040=ORIENTED_EDGE ( 'NONE', *, *, #26436, .F. ) ;
#37053=LINE ( 'NONE', #68045, #20900 ) ;
#37055=VERTEX_POINT ( 'NONE', #4424 ) ;
#37065=ORIENTED_EDGE ( 'NONE', *, *, #40417, .T. ) ;
#37088=EDGE_CURVE ( 'NONE', #8605, #24127, #64546, .T. ) ;
#37115=LINE ( 'NONE', #31840, #28748 ) ;
#37117=VERTEX_POINT ( 'NONE', #16354 ) ;
#37135=VECTOR ( 'NONE', #9089, 1000.000000000000000 ) ;
#37146=FACE_BOUND ( 'NONE', #62101, .T. ) ;
#37153=VERTEX_POINT ( 'NONE', #32881 ) ;
#37167=PLANE ( 'NONE',  #67773 ) ;
#37172=CARTESIAN_POINT ( 'NONE',  ( 15.55634918610406103, 15.55634918610400241, 0.000000000000000000 ) ) ;
#37177=ORIENTED_EDGE ( 'NONE', *, *, #63155, .F. ) ;
#37228=EDGE_CURVE ( 'NONE', #23144, #5719, #53629, .T. ) ;
#37240=ORIENTED_EDGE ( 'NONE', *, *, #19296, .F. ) ;
#37264=DIRECTION ( 'NONE',  ( 0.000000000000000000, 0.000000000000000000, 1.000000000000000000 ) ) ;
#37276=ORIENTED_EDGE ( 'NONE', *, *, #33922, .T. ) ;
#37282=EDGE_CURVE ( 'NONE', #8542, #47295, #22675, .T. ) ;
#37283=DIRECTION ( 'NONE',  ( 0.000000000000000000, 0.000000000000000000, 1.000000000000000000 ) ) ;
#37296=EDGE_CURVE ( 'NONE', #4563, #53791, #53961, .T. ) ;
#37301=EDGE_LOOP ( 'NONE', ( #41339, #12179, #58527, #34909 ) ) ;
#37313=DIRECTION ( 'NONE',  ( -1.000000000000000000, 0.000000000000000000, 0.000000000000000000 ) ) ;
#37323=EDGE_CURVE ( 'NONE', #48044, #16146, #8597, .T. ) ;
#37375=DIRECTION ( 'NONE',  ( 0.000000000000000000, 0.000000000000000000, -1.000000000000000000 ) ) ;
#37379=CARTESIAN_POINT ( 'NONE',  ( -15.55634918610403439, 0.000000000000000000, 0.000000000000000000 ) ) ;
#37396=CARTESIAN_POINT ( 'NONE',  ( 15.55634918610397399, -26.11269837220809364, 2.000000000000001776 ) ) ;
#37400=DIRECTION ( 'NONE',  ( 0.000000000000000000, 0.000000000000000000, -1.000000000000000000 ) ) ;
#37414=ADVANCED_FACE ( 'NONE', ( #26144 ), #68033, .F. ) ;
#37443=SHAPE_REPRESENTATION_RELATIONSHIP ( 'NONE' , 'NONE' ,  #36585, #61784 ) ;
#37449=CARTESIAN_POINT ( 'NONE',  ( 10.55634918610409656, 36.11269837220803680, 85.00100000000000477 ) ) ;
#37457=DIRECTION ( 'NONE',  ( 0.000000000000000000, -1.000000000000000000, 0.000000000000000000 ) ) ;
#37460=ORIENTED_EDGE ( 'NONE', *, *, #69237, .F. ) ;
#37466=VECTOR ( 'NONE', #26490, 1000.000000000000000 ) ;
#37487=FACE_OUTER_BOUND ( 'NONE', #7988, .T. ) ;
#37516=CIRCLE ( 'NONE', #7206, 54.99999999999995026 ) ;
#37523=VECTOR ( 'NONE', #4106, 1000.000000000000000 ) ;
#37525=LINE ( 'NONE', #5516, #29591 ) ;
#37528=DIRECTION ( 'NONE',  ( 1.000000000000000000, 0.000000000000000000, 0.000000000000000000 ) ) ;
#37537=DIRECTION ( 'NONE',  ( 1.000000000000000000, 0.000000000000000000, 0.000000000000000000 ) ) ;
#37548=LINE ( 'NONE', #16781, #35170 ) ;
#37571=DIRECTION ( 'NONE',  ( 1.000000000000000000, -0.000000000000000000, 0.000000000000000000 ) ) ;
#37605=VECTOR ( 'NONE', #26092, 1000.000000000000000 ) ;
#37611=VECTOR ( 'NONE', #59940, 1000.000000000000000 ) ;
#37650=EDGE_LOOP ( 'NONE', ( #23564, #12583, #65016, #10034 ) ) ;
#37669=DIRECTION ( 'NONE',  ( -0.000000000000000000, -0.000000000000000000, 1.000000000000000000 ) ) ;
#37672=DIRECTION ( 'NONE',  ( 0.000000000000000000, 1.000000000000000000, 0.000000000000000000 ) ) ;
#37679=PLANE ( 'NONE',  #51695 ) ;
#37700=ORIENTED_EDGE ( 'NONE', *, *, #55423, .F. ) ;
#37706=AXIS2_PLACEMENT_3D ( 'NONE', #37013, #42956, #25439 ) ;
#37709=VERTEX_POINT ( 'NONE', #13772 ) ;
#37734=LINE ( 'NONE', #52859, #60612 ) ;
#37737=ORIENTED_EDGE ( 'NONE', *, *, #66345, .F. ) ;
#37780=DIRECTION ( 'NONE',  ( -0.000000000000000000, -0.000000000000000000, -1.000000000000000000 ) ) ;
#37796=ORIENTED_EDGE ( 'NONE', *, *, #61227, .T. ) ;
#37818=ORIENTED_EDGE ( 'NONE', *, *, #33510, .T. ) ;
#37820=DIRECTION ( 'NONE',  ( 0.000000000000000000, -1.000000000000000000, 0.000000000000000000 ) ) ;
#37830=DIRECTION ( 'NONE',  ( -0.000000000000000000, -0.000000000000000000, -1.000000000000000000 ) ) ;
#37839=DIRECTION ( 'NONE',  ( 0.000000000000000000, 0.000000000000000000, -1.000000000000000000 ) ) ;
#37852=AXIS2_PLACEMENT_3D ( 'NONE', #11299, #54200, #6023 ) ;
#37873=EDGE_CURVE ( 'NONE', #59178, #36560, #64371, .T. ) ;
#37881=DIRECTION ( 'NONE',  ( -0.000000000000000000, -0.000000000000000000, -1.000000000000000000 ) ) ;
#37886=CARTESIAN_POINT ( 'NONE',  ( 15.55634918610396511, -46.66904755831214402, 0.000000000000000000 ) ) ;
#37887=ORIENTED_EDGE ( 'NONE', *, *, #52804, .T. ) ;
#37892=CARTESIAN_POINT ( 'NONE',  ( 31.11269837220812562, 36.11269837220800838, 2.000000000000001776 ) ) ;
#37911=AXIS2_PLACEMENT_3D ( 'NONE', #26732, #53096, #58385 ) ;
#37913=ORIENTED_EDGE ( 'NONE', *, *, #33180, .T. ) ;
#37914=DIRECTION ( 'NONE',  ( 0.000000000000000000, -1.000000000000000000, 0.000000000000000000 ) ) ;
#37949=ORIENTED_EDGE ( 'NONE', *, *, #34175, .F. ) ;
#37954=EDGE_CURVE ( 'NONE', #49516, #11433, #64036, .T. ) ;
#37961=DIRECTION ( 'NONE',  ( -0.000000000000000000, -0.000000000000000000, -1.000000000000000000 ) ) ;
#37965=VECTOR ( 'NONE', #33972, 1000.000000000000000 ) ;
#37982=ORIENTED_EDGE ( 'NONE', *, *, #33358, .T. ) ;
#37986=LINE ( 'NONE', #5285, #55402 ) ;
#37997=CARTESIAN_POINT ( 'NONE',  ( -5.000000000000000000, 0.000000000000000000, 2.000000000000000000 ) ) ;
#38009=DIRECTION ( 'NONE',  ( 1.000000000000000000, -0.000000000000000000, -0.000000000000000000 ) ) ;
#38018=DIRECTION ( 'NONE',  ( 0.000000000000000000, 1.000000000000000000, 0.000000000000000000 ) ) ;
#38028=CARTESIAN_POINT ( 'NONE',  ( 10.55634918610400419, -15.55634918610406103, 2.000000000000000000 ) ) ;
#38045=PLANE ( 'NONE',  #37852 ) ;
#38069=VERTEX_POINT ( 'NONE', #43608 ) ;
#38070=PLANE ( 'NONE',  #54865 ) ;
#38114=ORIENTED_EDGE ( 'NONE', *, *, #64306, .F. ) ;
#38116=ORIENTED_EDGE ( 'NONE', *, *, #48990, .F. ) ;
#38122=AXIS2_PLACEMENT_3D ( 'NONE', #43890, #17516, #55146 ) ;
#38137=CARTESIAN_POINT ( 'NONE',  ( 26.11269837220803325, -15.55634918610409656, 0.000000000000000000 ) ) ;
#38158=ADVANCED_FACE ( 'NONE', ( #34479, #23566 ), #49933, .T. ) ;
#38160=CARTESIAN_POINT ( 'NONE',  ( 0.000000000000000000, 0.000000000000000000, 15.70156211871650775 ) ) ;
#38179=ORIENTED_EDGE ( 'NONE', *, *, #51126, .T. ) ;
#38181=FACE_BOUND ( 'NONE', #37650, .T. ) ;
#38183=EDGE_CURVE ( 'NONE', #57137, #26420, #18282, .T. ) ;
#38198=FACE_OUTER_BOUND ( 'NONE', #55039, .T. ) ;
#38213=PLANE ( 'NONE',  #21318 ) ;
#38242=CARTESIAN_POINT ( 'NONE',  ( 15.55634918610397399, -31.11269837220809364, 85.00100000000000477 ) ) ;
#38252=LINE ( 'NONE', #11508, #25624 ) ;
#38283=DIRECTION ( 'NONE',  ( -1.000000000000000000, 0.000000000000000000, 0.000000000000000000 ) ) ;
#38288=FACE_OUTER_BOUND ( 'NONE', #588, .T. ) ;
#38292=DIRECTION ( 'NONE',  ( -0.000000000000000000, -0.000000000000000000, -1.000000000000000000 ) ) ;
#38304=LINE ( 'NONE', #16507, #12446 ) ;
#38328=EDGE_CURVE ( 'NONE', #59151, #35681, #24613, .T. ) ;
#38336=ORIENTED_EDGE ( 'NONE', *, *, #68683, .F. ) ;
#38337=ORIENTED_EDGE ( 'NONE', *, *, #8812, .F. ) ;
#38372=VECTOR ( 'NONE', #51603, 1000.000000000000000 ) ;
#38380=AXIS2_PLACEMENT_3D ( 'NONE', #35362, #56118, #40979 ) ;
#38392=CARTESIAN_POINT ( 'NONE',  ( 26.11269837220800127, -31.11269837220812562, 85.00100000000000477 ) ) ;
#38401=LINE ( 'NONE', #1467, #25440 ) ;
#38415=ADVANCED_FACE ( 'NONE', ( #20696 ), #21726, .F. ) ;
#38420=DIRECTION ( 'NONE',  ( 0.000000000000000000, 0.000000000000000000, 1.000000000000000000 ) ) ;
#38426=CARTESIAN_POINT ( 'NONE',  ( -15.55634918610405748, -10.55634918610400597, 2.000000000000001776 ) ) ;
#38443=AXIS2_PLACEMENT_3D ( 'NONE', #25228, #47342, #31195 ) ;
#38454=DIRECTION ( 'NONE',  ( 0.000000000000000000, 1.000000000000000000, -0.000000000000000000 ) ) ;
#38458=ORIENTED_EDGE ( 'NONE', *, *, #54565, .T. ) ;
#38463=DIRECTION ( 'NONE',  ( 0.000000000000000000, -1.000000000000000000, 0.000000000000000000 ) ) ;
#38482=VERTEX_POINT ( 'NONE', #55124 ) ;
#38503=DIRECTION ( 'NONE',  ( 0.000000000000000000, 1.000000000000000000, 0.000000000000000000 ) ) ;
#38506=LINE ( 'NONE', #65602, #32046 ) ;
#38507=LINE ( 'NONE', #6142, #53661 ) ;
#38519=VERTEX_POINT ( 'NONE', #20270 ) ;
#38528=VERTEX_POINT ( 'NONE', #19227 ) ;
#38538=VECTOR ( 'NONE', #66370, 1000.000000000000000 ) ;
#38550=ORIENTED_EDGE ( 'NONE', *, *, #59382, .T. ) ;
#38551=VERTEX_POINT ( 'NONE', #13613 ) ;
#38556=CARTESIAN_POINT ( 'NONE',  ( 31.11269837220809364, 15.55634918610396866, 2.000000000000001776 ) ) ;
#38559=DIRECTION ( 'NONE',  ( 0.000000000000000000, 0.000000000000000000, 1.000000000000000000 ) ) ;
#38564=ORIENTED_EDGE ( 'NONE', *, *, #22627, .F. ) ;
#38569=CARTESIAN_POINT ( 'NONE',  ( -15.55634918610411077, -46.66904755831208718, 2.000000000000001776 ) ) ;
#38576=CARTESIAN_POINT ( 'NONE',  ( -5.000000000000000000, 0.000000000000000000, 85.00100000000000477 ) ) ;
#38581=DIRECTION ( 'NONE',  ( 1.000000000000000000, 0.000000000000000000, 0.000000000000000000 ) ) ;
#38582=CARTESIAN_POINT ( 'NONE',  ( 15.55634918610409656, 31.11269837220803325, 85.00100000000000477 ) ) ;
#38594=EDGE_CURVE ( 'NONE', #913, #8504, #67783, .T. ) ;
#38607=LINE ( 'NONE', #7989, #26706 ) ;
#38614=ORIENTED_EDGE ( 'NONE', *, *, #65252, .F. ) ;
#38638=VERTEX_POINT ( 'NONE', #40682 ) ;
#38647=LINE ( 'NONE', #48470, #32811 ) ;
#38652=CARTESIAN_POINT ( 'NONE',  ( -36.11269837220804391, 15.55634918610408945, 85.00100000000000477 ) ) ;
#38654=ORIENTED_EDGE ( 'NONE', *, *, #40988, .T. ) ;
#38681=LINE ( 'NONE', #41806, #5373 ) ;
#38690=VECTOR ( 'NONE', #52957, 1000.000000000000000 ) ;
#38694=ORIENTED_EDGE ( 'NONE', *, *, #39300, .T. ) ;
#38704=PLANE ( 'NONE',  #49610 ) ;
#38705=ORIENTED_EDGE ( 'NONE', *, *, #12189, .T. ) ;
#38725=CARTESIAN_POINT ( 'NONE',  ( 10.55634918610406281, 20.55634918610400064, 85.00100000000000477 ) ) ;
#38726=ORIENTED_EDGE ( 'NONE', *, *, #6103, .T. ) ;
#38746=ORIENTED_EDGE ( 'NONE', *, *, #1768, .T. ) ;
#38756=ORIENTED_EDGE ( 'NONE', *, *, #17570, .T. ) ;
#38764=CARTESIAN_POINT ( 'NONE',  ( 15.55634918610400241, -10.55634918610406281, 85.00100000000000477 ) ) ;
#38765=EDGE_CURVE ( 'NONE', #53581, #50424, #13107, .T. ) ;
#38769=EDGE_CURVE ( 'NONE', #21122, #64911, #2545, .T. ) ;
#38815=VERTEX_POINT ( 'NONE', #45446 ) ;
#38817=VERTEX_POINT ( 'NONE', #39826 ) ;
#38876=CARTESIAN_POINT ( 'NONE',  ( -36.11269837220806522, 0.000000000000000000, 2.000000000000000000 ) ) ;
#38879=VECTOR ( 'NONE', #41165, 1000.000000000000000 ) ;
#38882=CARTESIAN_POINT ( 'NONE',  ( -15.55634918610403439, 5.000000000000028422, 0.000000000000000000 ) ) ;
#38937=LINE ( 'NONE', #28014, #44498 ) ;
#38938=VECTOR ( 'NONE', #13581, 1000.000000000000000 ) ;
#38982=EDGE_LOOP ( 'NONE', ( #11830, #15151, #67102, #68483 ) ) ;
#39015=DIRECTION ( 'NONE',  ( 0.000000000000000000, 1.000000000000000000, -0.000000000000000000 ) ) ;
#39019=EDGE_CURVE ( 'NONE', #38482, #32583, #60148, .T. ) ;
#39022=LINE ( 'NONE', #50262, #64795 ) ;
#39026=EDGE_LOOP ( 'NONE', ( #12048, #14249, #64102, #39850 ) ) ;
#39037=AXIS2_PLACEMENT_3D ( 'NONE', #6529, #65986, #37839 ) ;
#39049=ORIENTED_EDGE ( 'NONE', *, *, #4701, .T. ) ;
#39053=FACE_OUTER_BOUND ( 'NONE', #64205, .T. ) ;
#39057=EDGE_CURVE ( 'NONE', #57934, #21309, #28137, .T. ) ;
#39068=VECTOR ( 'NONE', #18811, 1000.000000000000000 ) ;
#39082=FACE_OUTER_BOUND ( 'NONE', #16114, .T. ) ;
#39084=DIRECTION ( 'NONE',  ( -1.000000000000000000, 0.000000000000000000, 0.000000000000000000 ) ) ;
#39101=VECTOR ( 'NONE', #62876, 1000.000000000000000 ) ;
#39103=VERTEX_POINT ( 'NONE', #34829 ) ;
#39117=ORIENTED_EDGE ( 'NONE', *, *, #56296, .T. ) ;
#39127=CARTESIAN_POINT ( 'NONE',  ( 31.11269837220800127, -31.11269837220812562, 0.000000000000000000 ) ) ;
#39137=CARTESIAN_POINT ( 'NONE',  ( 0.000000000000000000, 5.000000000000000000, 0.000000000000000000 ) ) ;
#39152=ORIENTED_EDGE ( 'NONE', *, *, #13497, .T. ) ;
#39164=CARTESIAN_POINT ( 'NONE',  ( 15.55634918610396511, -46.66904755831214402, 0.000000000000000000 ) ) ;
#39168=CARTESIAN_POINT ( 'NONE',  ( -5.000000000000026645, -15.55634918610403616, 2.000000000000000000 ) ) ;
#39177=LINE ( 'NONE', #56041, #25402 ) ;
#39202=LINE ( 'NONE', #2265, #26139 ) ;
#39205=CARTESIAN_POINT ( 'NONE',  ( 31.11269837220800127, -26.11269837220812562, 85.00100000000000477 ) ) ;
#39209=CARTESIAN_POINT ( 'NONE',  ( -31.11269837220812207, -31.11269837220801193, 85.00100000000000477 ) ) ;
#39217=CARTESIAN_POINT ( 'NONE',  ( -5.000000000000073719, -46.66904755831211560, 0.000000000000000000 ) ) ;
#39232=VECTOR ( 'NONE', #52966, 1000.000000000000000 ) ;
#39243=ADVANCED_FACE ( 'NONE', ( #48737 ), #33297, .F. ) ;
#39260=CARTESIAN_POINT ( 'NONE',  ( -36.11269837220801548, 31.11269837220812207, 0.000000000000000000 ) ) ;
#39282=VECTOR ( 'NONE', #8273, 1000.000000000000000 ) ;
#39300=EDGE_CURVE ( 'NONE', #30808, #40134, #35285, .T. ) ;
#39313=EDGE_CURVE ( 'NONE', #32720, #56407, #49793, .T. ) ;
#39317=DIRECTION ( 'NONE',  ( 0.000000000000000000, 1.000000000000000000, -0.000000000000000000 ) ) ;
#39330=FACE_BOUND ( 'NONE', #52835, .T. ) ;
#39331=VERTEX_POINT ( 'NONE', #15893 ) ;
#39337=ORIENTED_EDGE ( 'NONE', *, *, #31587, .F. ) ;
#39346=DIRECTION ( 'NONE',  ( -1.000000000000000000, 0.000000000000000000, 0.000000000000000000 ) ) ;
#39380=CARTESIAN_POINT ( 'NONE',  ( -5.767955557622883589E-14, -31.11269837220806878, 2.000000000000001776 ) ) ;
#39387=LINE ( 'NONE', #28480, #31298 ) ;
#39410=DIRECTION ( 'NONE',  ( 0.000000000000000000, 1.000000000000000000, 0.000000000000000000 ) ) ;
#39428=CARTESIAN_POINT ( 'NONE',  ( -31.11269837220804035, 15.55634918610408945, 0.000000000000000000 ) ) ;
#39436=DIRECTION ( 'NONE',  ( 1.000000000000000000, -0.000000000000000000, 0.000000000000000000 ) ) ;
#39440=DIRECTION ( 'NONE',  ( -0.000000000000000000, -1.000000000000000000, -0.000000000000000000 ) ) ;
#39445=ORIENTED_EDGE ( 'NONE', *, *, #58330, .F. ) ;
#39452=ADVANCED_FACE ( 'NONE', ( #16236 ), #42286, .F. ) ;
#39461=CARTESIAN_POINT ( 'NONE',  ( -15.55634918610396866, 31.11269837220809009, 0.000000000000000000 ) ) ;
#39473=ORIENTED_EDGE ( 'NONE', *, *, #19296, .T. ) ;
#39476=ORIENTED_EDGE ( 'NONE', *, *, #19380, .T. ) ;
#39485=VECTOR ( 'NONE', #50109, 1000.000000000000000 ) ;
#39496=ORIENTED_EDGE ( 'NONE', *, *, #234, .F. ) ;
#39508=ORIENTED_EDGE ( 'NONE', *, *, #54789, .T. ) ;
#39519=VERTEX_POINT ( 'NONE', #32426 ) ;
#39544=LINE ( 'NONE', #39205, #34927 ) ;
#39562=FACE_OUTER_BOUND ( 'NONE', #67114, .T. ) ;
#39582=EDGE_CURVE ( 'NONE', #55128, #62781, #49986, .T. ) ;
#39607=LINE ( 'NONE', #61742, #67234 ) ;
#39614=ORIENTED_EDGE ( 'NONE', *, *, #16669, .F. ) ;
#39632=ADVANCED_FACE ( 'NONE', ( #60190 ), #33482, .F. ) ;
#39680=VERTEX_POINT ( 'NONE', #66196 ) ;
#39681=VERTEX_POINT ( 'NONE', #17989 ) ;
#39698=EDGE_LOOP ( 'NONE', ( #6976, #46148, #42257, #48987 ) ) ;
#39700=EDGE_CURVE ( 'NONE', #38482, #18908, #2162, .T. ) ;
#39724=ORIENTED_EDGE ( 'NONE', *, *, #68839, .F. ) ;
#39729=DIRECTION ( 'NONE',  ( 0.000000000000000000, -1.000000000000000000, 0.000000000000000000 ) ) ;
#39738=VECTOR ( 'NONE', #53080, 1000.000000000000000 ) ;
#39741=LINE ( 'NONE', #44311, #26293 ) ;
#39746=VECTOR ( 'NONE', #22677, 1000.000000000000000 ) ;
#39751=VECTOR ( 'NONE', #48604, 1000.000000000000000 ) ;
#39765=EDGE_LOOP ( 'NONE', ( #48662, #16821, #15305, #40563 ) ) ;
#39800=LINE ( 'NONE', #50357, #24236 ) ;
#39806=EDGE_CURVE ( 'NONE', #50609, #23032, #61592, .T. ) ;
#39824=DIRECTION ( 'NONE',  ( 0.000000000000000000, -1.000000000000000000, 0.000000000000000000 ) ) ;
#39826=CARTESIAN_POINT ( 'NONE',  ( -31.11269837220801193, 31.11269837220812207, 0.000000000000000000 ) ) ;
#39845=DIRECTION ( 'NONE',  ( -0.000000000000000000, -0.000000000000000000, -1.000000000000000000 ) ) ;
#39850=ORIENTED_EDGE ( 'NONE', *, *, #50642, .T. ) ;
#39864=EDGE_LOOP ( 'NONE', ( #34025, #38116, #60982, #34442 ) ) ;
#39872=DIRECTION ( 'NONE',  ( -0.000000000000000000, -0.000000000000000000, -1.000000000000000000 ) ) ;
#39883=EDGE_CURVE ( 'NONE', #38638, #29482, #27388, .T. ) ;
#39887=CARTESIAN_POINT ( 'NONE',  ( 10.55634918610397577, -31.11269837220809364, 0.000000000000000000 ) ) ;
#39888=AXIS2_PLACEMENT_3D ( 'NONE', #41253, #2924, #24037 ) ;
#39909=DIRECTION ( 'NONE',  ( 1.000000000000000000, -0.000000000000000000, 0.000000000000000000 ) ) ;
#39911=ORIENTED_EDGE ( 'NONE', *, *, #62681, .T. ) ;
#39914=PLANE ( 'NONE',  #53753 ) ;
#39994=DIRECTION ( 'NONE',  ( -0.000000000000000000, -0.000000000000000000, -1.000000000000000000 ) ) ;
#40018=FACE_BOUND ( 'NONE', #2482, .T. ) ;
#40027=ADVANCED_FACE ( 'NONE', ( #18589 ), #55883, .F. ) ;
#40039=LINE ( 'NONE', #34772, #1090 ) ;
#40048=ORIENTED_EDGE ( 'NONE', *, *, #54686, .F. ) ;
#40060=EDGE_LOOP ( 'NONE', ( #20872, #63405, #33413, #18555 ) ) ;
#40063=DIRECTION ( 'NONE',  ( -0.000000000000000000, -0.000000000000000000, -1.000000000000000000 ) ) ;
#40090=CARTESIAN_POINT ( 'NONE',  ( 7.762887554996211747E-14, 46.66904755831208718, 0.000000000000000000 ) ) ;
#40092=ORIENTED_EDGE ( 'NONE', *, *, #52807, .T. ) ;
#40094=EDGE_CURVE ( 'NONE', #30890, #19565, #14691, .T. ) ;
#40128=FACE_OUTER_BOUND ( 'NONE', #66244, .T. ) ;
#40129=FACE_OUTER_BOUND ( 'NONE', #51563, .T. ) ;
#40132=VECTOR ( 'NONE', #44724, 1000.000000000000000 ) ;
#40134=VERTEX_POINT ( 'NONE', #10442 ) ;
#40148=CARTESIAN_POINT ( 'NONE',  ( -31.11269837220809364, -15.55634918610397754, 2.000000000000001776 ) ) ;
#40154=CARTESIAN_POINT ( 'NONE',  ( -51.66904755831210139, 6.635317295611287136E-14, 2.000000000000001776 ) ) ;
#40160=LINE ( 'NONE', #28203, #344 ) ;
#40169=EDGE_CURVE ( 'NONE', #14795, #5765, #48070, .T. ) ;
#40190=VECTOR ( 'NONE', #20531, 1000.000000000000000 ) ;
#40198=CARTESIAN_POINT ( 'NONE',  ( -46.66904755831210139, 6.635317295611287136E-14, 85.00100000000000477 ) ) ;
#40217=ORIENTED_EDGE ( 'NONE', *, *, #67129, .F. ) ;
#40219=CARTESIAN_POINT ( 'NONE',  ( -15.55634918610400597, 15.55634918610405748, 0.000000000000000000 ) ) ;
#40237=ORIENTED_EDGE ( 'NONE', *, *, #53979, .F. ) ;
#40261=DIRECTION ( 'NONE',  ( 0.000000000000000000, 1.000000000000000000, 0.000000000000000000 ) ) ;
#40273=VERTEX_POINT ( 'NONE', #24496 ) ;
#40281=AXIS2_PLACEMENT_3D ( 'NONE', #59607, #33609, #11781 ) ;
#40290=LINE ( 'NONE', #1608, #60150 ) ;
#40301=CARTESIAN_POINT ( 'NONE',  ( 41.66904755831210849, -9.150666335777657423E-14, 0.000000000000000000 ) ) ;
#40304=DIRECTION ( 'NONE',  ( -1.000000000000000000, 0.000000000000000000, 0.000000000000000000 ) ) ;
#40307=ORIENTED_EDGE ( 'NONE', *, *, #234, .T. ) ;
#40328=ORIENTED_EDGE ( 'NONE', *, *, #27929, .T. ) ;
#40336=EDGE_CURVE ( 'NONE', #44250, #61065, #1635, .T. ) ;
#40389=CARTESIAN_POINT ( 'NONE',  ( 10.55634918610409656, 31.11269837220803325, 2.000000000000000000 ) ) ;
#40392=CARTESIAN_POINT ( 'NONE',  ( 41.66904755831212981, 20.55634918610394379, 85.00100000000000477 ) ) ;
#40417=EDGE_CURVE ( 'NONE', #27957, #25366, #19898, .T. ) ;
#40418=LINE ( 'NONE', #41469, #1007 ) ;
#40433=EDGE_LOOP ( 'NONE', ( #22336, #19691, #32778, #47601 ) ) ;
#40435=ORIENTED_EDGE ( 'NONE', *, *, #19770, .T. ) ;
#40439=ORIENTED_EDGE ( 'NONE', *, *, #7943, .F. ) ;
#40502=ORIENTED_EDGE ( 'NONE', *, *, #32277, .T. ) ;
#40521=ORIENTED_EDGE ( 'NONE', *, *, #8963, .T. ) ;
#40547=PLANE ( 'NONE',  #33161 ) ;
#40551=ORIENTED_EDGE ( 'NONE', *, *, #7740, .F. ) ;
#40563=ORIENTED_EDGE ( 'NONE', *, *, #1009, .F. ) ;
#40566=DIRECTION ( 'NONE',  ( 0.000000000000000000, 1.000000000000000000, -0.000000000000000000 ) ) ;
#40592=DIRECTION ( 'NONE',  ( 0.000000000000000000, -1.000000000000000000, 0.000000000000000000 ) ) ;
#40593=AXIS2_PLACEMENT_3D ( 'NONE', #68128, #30831, #14644 ) ;
#40599=ORIENTED_EDGE ( 'NONE', *, *, #26208, .T. ) ;
#40602=CARTESIAN_POINT ( 'NONE',  ( 10.55634918610403084, 4.999999999999969802, 0.000000000000000000 ) ) ;
#40607=VECTOR ( 'NONE', #37780, 1000.000000000000000 ) ;
#40630=ORIENTED_EDGE ( 'NONE', *, *, #43838, .T. ) ;
#40652=VECTOR ( 'NONE', #9479, 1000.000000000000000 ) ;
#40662=LINE ( 'NONE', #35395, #10647 ) ;
#40677=LINE ( 'NONE', #36107, #12482 ) ;
#40682=CARTESIAN_POINT ( 'NONE',  ( -7.329206686002009974E-14, -41.66904755831212270, 0.000000000000000000 ) ) ;
#40693=EDGE_LOOP ( 'NONE', ( #16332, #46241, #48461, #68589 ) ) ;
#40701=FACE_BOUND ( 'NONE', #68225, .T. ) ;
#40729=DIRECTION ( 'NONE',  ( -1.000000000000000000, 0.000000000000000000, 0.000000000000000000 ) ) ;
#40731=DIRECTION ( 'NONE',  ( -1.000000000000000000, 0.000000000000000000, 0.000000000000000000 ) ) ;
#40735=DIRECTION ( 'NONE',  ( -0.000000000000000000, -0.000000000000000000, -1.000000000000000000 ) ) ;
#40742=CARTESIAN_POINT ( 'NONE',  ( -15.55634918610400597, 20.55634918610405748, 2.000000000000001776 ) ) ;
#40747=VERTEX_POINT ( 'NONE', #58464 ) ;
#40781=AXIS2_PLACEMENT_3D ( 'NONE', #32076, #20827, #26109 ) ;
#40791=VECTOR ( 'NONE', #43854, 1000.000000000000000 ) ;
#40797=AXIS2_PLACEMENT_3D ( 'NONE', #39209, #12126, #7552 ) ;
#40815=ADVANCED_FACE ( 'NONE', ( #54834 ), #49907, .F. ) ;
#40853=VERTEX_POINT ( 'NONE', #24592 ) ;
#40863=CARTESIAN_POINT ( 'NONE',  ( -46.66904755831212981, -15.55634918610397222, 85.00100000000000477 ) ) ;
#40879=DIRECTION ( 'NONE',  ( 0.000000000000000000, 1.000000000000000000, -0.000000000000000000 ) ) ;
#40899=ORIENTED_EDGE ( 'NONE', *, *, #42450, .T. ) ;
#40905=ORIENTED_EDGE ( 'NONE', *, *, #16012, .T. ) ;
#40914=LINE ( 'NONE', #45489, #20297 ) ;
#40945=ORIENTED_EDGE ( 'NONE', *, *, #46393, .T. ) ;
#40953=CARTESIAN_POINT ( 'NONE',  ( 10.55634918610406281, 20.55634918610400064, 2.000000000000001776 ) ) ;
#40964=ADVANCED_FACE ( 'NONE', ( #60392 ), #16436, .F. ) ;
#40965=ORIENTED_EDGE ( 'NONE', *, *, #48455, .T. ) ;
#40968=DIRECTION ( 'NONE',  ( -1.000000000000000000, 0.000000000000000000, 0.000000000000000000 ) ) ;
#40979=DIRECTION ( 'NONE',  ( 0.000000000000000000, 0.000000000000000000, 1.000000000000000000 ) ) ;
#40988=EDGE_CURVE ( 'NONE', #11058, #39519, #34059, .T. ) ;
#41014=EDGE_LOOP ( 'NONE', ( #4933, #16317, #53691, #18377 ) ) ;
#41022=VERTEX_POINT ( 'NONE', #37892 ) ;
#41031=DIRECTION ( 'NONE',  ( 0.000000000000000000, 0.000000000000000000, -1.000000000000000000 ) ) ;
#41062=CARTESIAN_POINT ( 'NONE',  ( 41.66904755831208007, -15.55634918610412853, 85.00100000000000477 ) ) ;
#41073=CARTESIAN_POINT ( 'NONE',  ( 15.55634918610396511, -41.66904755831214402, 85.00100000000000477 ) ) ;
#41086=CARTESIAN_POINT ( 'NONE',  ( -31.11269837220812207, -31.11269837220801193, 2.000000000000001776 ) ) ;
#41097=AXIS2_PLACEMENT_3D ( 'NONE', #11685, #32115, #37375 ) ;
#41115=CARTESIAN_POINT ( 'NONE',  ( 0.000000000000000000, 0.000000000000000000, 85.00000000000000000 ) ) ;
#41118=EDGE_CURVE ( 'NONE', #15890, #22095, #45943, .T. ) ;
#41148=CARTESIAN_POINT ( 'NONE',  ( 31.11269837220800127, -31.11269837220812562, 0.000000000000000000 ) ) ;
#41150=VECTOR ( 'NONE', #39440, 1000.000000000000000 ) ;
#41159=ORIENTED_EDGE ( 'NONE', *, *, #54955, .T. ) ;
#41162=DIRECTION ( 'NONE',  ( -1.000000000000000000, 0.000000000000000000, 0.000000000000000000 ) ) ;
#41165=DIRECTION ( 'NONE',  ( -1.000000000000000000, 0.000000000000000000, 0.000000000000000000 ) ) ;
#41176=CARTESIAN_POINT ( 'NONE',  ( 31.11269837220809364, 15.55634918610396866, 85.00100000000000477 ) ) ;
#41186=DIRECTION ( 'NONE',  ( -0.000000000000000000, -0.000000000000000000, -1.000000000000000000 ) ) ;
#41192=DIRECTION ( 'NONE',  ( -0.000000000000000000, -0.000000000000000000, -1.000000000000000000 ) ) ;
#41218=VERTEX_POINT ( 'NONE', #67757 ) ;
#41225=ADVANCED_FACE ( 'NONE', ( #50533 ), #30810, .F. ) ;
#41246=DIRECTION ( 'NONE',  ( 0.000000000000000000, 1.000000000000000000, -0.000000000000000000 ) ) ;
#41247=CARTESIAN_POINT ( 'NONE',  ( 15.55634918610406103, 15.55634918610400241, 85.00100000000000477 ) ) ;
#41251=LINE ( 'NONE', #68656, #14826 ) ;
#41253=CARTESIAN_POINT ( 'NONE',  ( -15.55634918610400597, 15.55634918610405748, 85.00100000000000477 ) ) ;
#41256=VECTOR ( 'NONE', #22632, 1000.000000000000000 ) ;
#41288=VECTOR ( 'NONE', #65324, 1000.000000000000000 ) ;
#41295=DIRECTION ( 'NONE',  ( 0.000000000000000000, -0.000000000000000000, -1.000000000000000000 ) ) ;
#41339=ORIENTED_EDGE ( 'NONE', *, *, #5567, .F. ) ;
#41341=ORIENTED_EDGE ( 'NONE', *, *, #51126, .F. ) ;
#41347=VECTOR ( 'NONE', #51701, 1000.000000000000000 ) ;
#41358=FACE_OUTER_BOUND ( 'NONE', #52412, .T. ) ;
#41365=ORIENTED_EDGE ( 'NONE', *, *, #12054, .T. ) ;
#41384=DIRECTION ( 'NONE',  ( -0.000000000000000000, -0.000000000000000000, -1.000000000000000000 ) ) ;
#41394=VECTOR ( 'NONE', #2113, 1000.000000000000000 ) ;
#41401=ORIENTED_EDGE ( 'NONE', *, *, #58585, .T. ) ;
#41411=PLANE ( 'NONE',  #20500 ) ;
#41414=ADVANCED_FACE ( 'NONE', ( #8235 ), #13171, .F. ) ;
#41422=LINE ( 'NONE', #47365, #39101 ) ;
#41430=VERTEX_POINT ( 'NONE', #51146 ) ;
#41444=VECTOR ( 'NONE', #58733, 1000.000000000000000 ) ;
#41452=PLANE ( 'NONE',  #67070 ) ;
#41454=EDGE_CURVE ( 'NONE', #11967, #40747, #12825, .T. ) ;
#41469=CARTESIAN_POINT ( 'NONE',  ( -7.329206686002009974E-14, -46.66904755831211560, 0.000000000000000000 ) ) ;
#41482=ORIENTED_EDGE ( 'NONE', *, *, #38183, .F. ) ;
#41525=LINE ( 'NONE', #30977, #65658 ) ;
#41528=ORIENTED_EDGE ( 'NONE', *, *, #29092, .F. ) ;
#41533=LINE ( 'NONE', #40154, #68944 ) ;
#41552=AXIS2_PLACEMENT_3D ( 'NONE', #28883, #33806, #1446 ) ;
#41602=DIRECTION ( 'NONE',  ( 0.000000000000000000, -1.000000000000000000, 0.000000000000000000 ) ) ;
#41605=EDGE_CURVE ( 'NONE', #36801, #55179, #29592, .T. ) ;
#41616=DIRECTION ( 'NONE',  ( 0.000000000000000000, 1.000000000000000000, -0.000000000000000000 ) ) ;
#41623=CARTESIAN_POINT ( 'NONE',  ( -31.11269837220806878, 5.594483210025202879E-14, 85.00100000000000477 ) ) ;
#41674=EDGE_CURVE ( 'NONE', #14714, #8542, #40160, .T. ) ;
#41676=ORIENTED_EDGE ( 'NONE', *, *, #51845, .F. ) ;
#41692=CARTESIAN_POINT ( 'NONE',  ( -15.55634918610396866, 31.11269837220809009, 2.000000000000001776 ) ) ;
#41695=EDGE_CURVE ( 'NONE', #63634, #58410, #13428, .T. ) ;
#41707=CARTESIAN_POINT ( 'NONE',  ( -65.00000000000000000, 7.960204194457797252E-15, -0.002000000000002000178 ) ) ;
#41710=VECTOR ( 'NONE', #46416, 1000.000000000000000 ) ;
#41718=ADVANCED_FACE ( 'NONE', ( #12383 ), #24018, .F. ) ;
#41729=ORIENTED_EDGE ( 'NONE', *, *, #35646, .T. ) ;
#41745=ORIENTED_EDGE ( 'NONE', *, *, #54960, .T. ) ;
#41753=VECTOR ( 'NONE', #49251, 1000.000000000000000 ) ;
#41786=CARTESIAN_POINT ( 'NONE',  ( -46.66904755831210139, 5.000000000000066613, 2.000000000000001776 ) ) ;
#41793=CARTESIAN_POINT ( 'NONE',  ( 72.99999999999998579, 8.939921633775675282E-15, 85.00000000000000000 ) ) ;
#41798=ORIENTED_EDGE ( 'NONE', *, *, #1915, .F. ) ;
#41802=CARTESIAN_POINT ( 'NONE',  ( -36.11269837220804391, 15.55634918610408945, 2.000000000000000000 ) ) ;
#41806=CARTESIAN_POINT ( 'NONE',  ( -15.55634918610396866, 31.11269837220809009, 85.00100000000000477 ) ) ;
#41807=VECTOR ( 'NONE', #4542, 1000.000000000000000 ) ;
#41811=VECTOR ( 'NONE', #59396, 1000.000000000000000 ) ;
#41858=FACE_OUTER_BOUND ( 'NONE', #44786, .T. ) ;
#41859=ORIENTED_EDGE ( 'NONE', *, *, #51773, .T. ) ;
#41865=DIRECTION ( 'NONE',  ( 1.000000000000000000, 0.000000000000000000, 0.000000000000000000 ) ) ;
#41880=VERTEX_POINT ( 'NONE', #50288 ) ;
#41901=VECTOR ( 'NONE', #52174, 1000.000000000000000 ) ;
#41905=ORIENTED_EDGE ( 'NONE', *, *, #14337, .T. ) ;
#41933=ORIENTED_EDGE ( 'NONE', *, *, #40988, .F. ) ;
#41942=CARTESIAN_POINT ( 'NONE',  ( -4.999999999999971578, 20.55634918610402906, 0.000000000000000000 ) ) ;
#41965=CARTESIAN_POINT ( 'NONE',  ( 7.762887554996211747E-14, 46.66904755831208718, 85.00100000000000477 ) ) ;
#41968=DIRECTION ( 'NONE',  ( -0.000000000000000000, -0.000000000000000000, -1.000000000000000000 ) ) ;
#41969=PLANE ( 'NONE',  #20952 ) ;
#41976=FACE_OUTER_BOUND ( 'NONE', #18761, .T. ) ;
#41990=VECTOR ( 'NONE', #26637, 1000.000000000000000 ) ;
#42014=LINE ( 'NONE', #20214, #27175 ) ;
#42033=VERTEX_POINT ( 'NONE', #54608 ) ;
#42040=VECTOR ( 'NONE', #40063, 1000.000000000000000 ) ;
#42061=ORIENTED_EDGE ( 'NONE', *, *, #23667, .T. ) ;
#42085=CARTESIAN_POINT ( 'NONE',  ( 41.66904755831212981, 15.55634918610394379, 85.00100000000000477 ) ) ;
#42116=ORIENTED_EDGE ( 'NONE', *, *, #52093, .F. ) ;
#42166=CARTESIAN_POINT ( 'NONE',  ( -7.329206686002009974E-14, -46.66904755831211560, 2.000000000000001776 ) ) ;
#42192=CARTESIAN_POINT ( 'NONE',  ( 31.11269837220812562, 31.11269837220800483, 0.000000000000000000 ) ) ;
#42209=CARTESIAN_POINT ( 'NONE',  ( 31.11269837220812562, 31.11269837220800483, 85.00100000000000477 ) ) ;
#42214=PLANE ( 'NONE',  #17236 ) ;
#42234=EDGE_CURVE ( 'NONE', #58547, #18138, #54872, .T. ) ;
#42254=ORIENTED_EDGE ( 'NONE', *, *, #56996, .T. ) ;
#42257=ORIENTED_EDGE ( 'NONE', *, *, #49791, .F. ) ;
#42270=LINE ( 'NONE', #3951, #37605 ) ;
#42272=CARTESIAN_POINT ( 'NONE',  ( -5.000000000000073719, -41.66904755831212270, 2.000000000000001776 ) ) ;
#42286=PLANE ( 'NONE',  #40781 ) ;
#42287=ORIENTED_EDGE ( 'NONE', *, *, #69237, .T. ) ;
#42290=DIRECTION ( 'NONE',  ( -0.000000000000000000, -0.000000000000000000, -1.000000000000000000 ) ) ;
#42295=CARTESIAN_POINT ( 'NONE',  ( -31.11269837220804035, 20.55634918610408945, 2.000000000000001776 ) ) ;
#42305=LINE ( 'NONE', #9953, #46501 ) ;
#42311=CARTESIAN_POINT ( 'NONE',  ( -20.55634918610411077, -46.66904755831208718, 0.000000000000000000 ) ) ;
#42333=CARTESIAN_POINT ( 'NONE',  ( 46.66904755831212981, 20.55634918610394379, 2.000000000000001776 ) ) ;
#42343=DIRECTION ( 'NONE',  ( 0.000000000000000000, 1.000000000000000000, 0.000000000000000000 ) ) ;
#42346=ORIENTED_EDGE ( 'NONE', *, *, #36691, .T. ) ;
#42376=EDGE_LOOP ( 'NONE', ( #53104, #11377, #24587, #13368 ) ) ;
#42408=VERTEX_POINT ( 'NONE', #65365 ) ;
#42450=EDGE_CURVE ( 'NONE', #56697, #6738, #50226, .T. ) ;
#42465=DIRECTION ( 'NONE',  ( -0.000000000000000000, -0.000000000000000000, 1.000000000000000000 ) ) ;
#42491=ORIENTED_EDGE ( 'NONE', *, *, #63382, .F. ) ;
#42509=CARTESIAN_POINT ( 'NONE',  ( -66.50000000000000000, 8.541911424052787628E-15, 17.57656211871651308 ) ) ;
#42510=ORIENTED_EDGE ( 'NONE', *, *, #36279, .F. ) ;
#42542=EDGE_LOOP ( 'NONE', ( #11884, #55325, #2550, #59002 ) ) ;
#42553=CARTESIAN_POINT ( 'NONE',  ( -15.55634918610403439, 5.000000000000028422, 85.00100000000000477 ) ) ;
#42560=DIRECTION ( 'NONE',  ( 0.000000000000000000, 0.000000000000000000, 1.000000000000000000 ) ) ;
#42561=EDGE_CURVE ( 'NONE', #5030, #15461, #15011, .T. ) ;
#42588=EDGE_CURVE ( 'NONE', #65715, #48270, #11798, .T. ) ;
#42593=CARTESIAN_POINT ( 'NONE',  ( -5.000000000000026645, -15.55634918610403616, 2.000000000000001776 ) ) ;
#42595=ORIENTED_EDGE ( 'NONE', *, *, #1164, .T. ) ;
#42602=CARTESIAN_POINT ( 'NONE',  ( 31.11269837220803325, -15.55634918610409656, 0.000000000000000000 ) ) ;
#42603=LINE ( 'NONE', #53829, #15439 ) ;
#42604=CARTESIAN_POINT ( 'NONE',  ( -51.66904755831210139, 6.635317295611287136E-14, 85.00100000000000477 ) ) ;
#42616=DIRECTION ( 'NONE',  ( -0.000000000000000000, -0.000000000000000000, -1.000000000000000000 ) ) ;
#42623=ORIENTED_EDGE ( 'NONE', *, *, #69086, .T. ) ;
#42631=AXIS2_PLACEMENT_3D ( 'NONE', #57559, #19574, #41031 ) ;
#42675=DIRECTION ( 'NONE',  ( 1.000000000000000000, 0.000000000000000000, 0.000000000000000000 ) ) ;
#42679=CARTESIAN_POINT ( 'NONE',  ( 10.55634918610409656, 31.11269837220803325, 0.000000000000000000 ) ) ;
#42683=CARTESIAN_POINT ( 'NONE',  ( 46.66904755831207297, -15.55634918610412853, 0.000000000000000000 ) ) ;
#42702=LINE ( 'NONE', #64158, #11558 ) ;
#42722=VECTOR ( 'NONE', #25909, 1000.000000000000000 ) ;
#42752=CARTESIAN_POINT ( 'NONE',  ( 15.55634918610411610, 51.66904755831205875, 0.000000000000000000 ) ) ;
#42753=VECTOR ( 'NONE', #21354, 1000.000000000000000 ) ;
#42755=DIRECTION ( 'NONE',  ( 0.000000000000000000, 0.000000000000000000, 1.000000000000000000 ) ) ;
#42760=FACE_BOUND ( 'NONE', #42376, .T. ) ;
#42767=CARTESIAN_POINT ( 'NONE',  ( -31.11269837220809364, -15.55634918610397754, 0.000000000000000000 ) ) ;
#42768=PLANE ( 'NONE',  #56973 ) ;
#42801=LINE ( 'NONE', #26975, #74 ) ;
#42846=ORIENTED_EDGE ( 'NONE', *, *, #67027, .T. ) ;
#42851=CARTESIAN_POINT ( 'NONE',  ( -15.55634918610396866, 31.11269837220809009, 0.000000000000000000 ) ) ;
#42874=CARTESIAN_POINT ( 'NONE',  ( 46.66904755831207297, -10.55634918610412853, 0.000000000000000000 ) ) ;
#42888=VECTOR ( 'NONE', #29055, 1000.000000000000000 ) ;
#42889=CARTESIAN_POINT ( 'NONE',  ( 31.11269837220803325, -10.55634918610409656, 2.000000000000001776 ) ) ;
#42890=CARTESIAN_POINT ( 'NONE',  ( 15.55634918610400241, -15.55634918610406103, 2.000000000000001776 ) ) ;
#42901=DIRECTION ( 'NONE',  ( -1.000000000000000000, 0.000000000000000000, 0.000000000000000000 ) ) ;
#42915=ORIENTED_EDGE ( 'NONE', *, *, #27694, .F. ) ;
#42918=EDGE_CURVE ( 'NONE', #47295, #38817, #56630, .T. ) ;
#42920=VERTEX_POINT ( 'NONE', #51363 ) ;
#42924=VECTOR ( 'NONE', #57338, 1000.000000000000000 ) ;
#42929=DIRECTION ( 'NONE',  ( 1.000000000000000000, -0.000000000000000000, 0.000000000000000000 ) ) ;
#42939=LINE ( 'NONE', #64408, #2736 ) ;
#42949=CARTESIAN_POINT ( 'NONE',  ( 41.66904755831210849, 0.000000000000000000, 2.000000000000000000 ) ) ;
#42951=ORIENTED_EDGE ( 'NONE', *, *, #19934, .F. ) ;
#42956=DIRECTION ( 'NONE',  ( 1.000000000000000000, 0.000000000000000000, 0.000000000000000000 ) ) ;
#42964=LINE ( 'NONE', #43311, #22972 ) ;
#42967=ORIENTED_EDGE ( 'NONE', *, *, #18590, .F. ) ;
#42991=DIRECTION ( 'NONE',  ( 0.000000000000000000, 1.000000000000000000, -0.000000000000000000 ) ) ;
#43017=EDGE_CURVE ( 'NONE', #30419, #64201, #22450, .T. ) ;
#43028=DIRECTION ( 'NONE',  ( -1.000000000000000000, 0.000000000000000000, 0.000000000000000000 ) ) ;
#43029=DIRECTION ( 'NONE',  ( -0.000000000000000000, -0.000000000000000000, -1.000000000000000000 ) ) ;
#43100=DIRECTION ( 'NONE',  ( 0.000000000000000000, 1.000000000000000000, -0.000000000000000000 ) ) ;
#43101=LINE ( 'NONE', #190, #29805 ) ;
#43105=FACE_BOUND ( 'NONE', #67926, .T. ) ;
#43108=EDGE_CURVE ( 'NONE', #4486, #54708, #7679, .T. ) ;
#43113=ORIENTED_EDGE ( 'NONE', *, *, #57336, .T. ) ;
#43120=CARTESIAN_POINT ( 'NONE',  ( -2.645453300864630819E-14, -15.55634918610403616, 85.00100000000000477 ) ) ;
#43125=DIRECTION ( 'NONE',  ( 1.000000000000000000, 0.000000000000000000, 0.000000000000000000 ) ) ;
#43128=CARTESIAN_POINT ( 'NONE',  ( -51.66904755831212981, -10.55634918610397222, 2.000000000000001776 ) ) ;
#43146=CARTESIAN_POINT ( 'NONE',  ( -15.55634918610405748, -15.55634918610400774, 2.000000000000001776 ) ) ;
#43194=CARTESIAN_POINT ( 'NONE',  ( -51.66904755831210139, 5.000000000000066613, 85.00100000000000477 ) ) ;
#43211=DIRECTION ( 'NONE',  ( -0.000000000000000000, -0.000000000000000000, -1.000000000000000000 ) ) ;
#43221=VECTOR ( 'NONE', #13562, 1000.000000000000000 ) ;
#43235=VECTOR ( 'NONE', #36551, 1000.000000000000000 ) ;
#43252=PLANE ( 'NONE',  #26288 ) ;
#43269=PLANE ( 'NONE',  #54115 ) ;
#43311=CARTESIAN_POINT ( 'NONE',  ( 46.66904755831207297, -15.55634918610412853, 85.00100000000000477 ) ) ;
#43324=VECTOR ( 'NONE', #60030, 1000.000000000000000 ) ;
#43332=PRODUCT_DEFINITION_FORMATION_WITH_SPECIFIED_SOURCE ( 'ANY', '', #56359, .NOT_KNOWN. ) ;
#43340=CARTESIAN_POINT ( 'NONE',  ( 26.11269837220800127, -31.11269837220812562, 2.000000000000001776 ) ) ;
#43349=CARTESIAN_POINT ( 'NONE',  ( -51.66904755831210139, 5.000000000000066613, 0.000000000000000000 ) ) ;
#43353=DIRECTION ( 'NONE',  ( 0.000000000000000000, 1.000000000000000000, -0.000000000000000000 ) ) ;
#43363=FACE_OUTER_BOUND ( 'NONE', #25776, .T. ) ;
#43364=CARTESIAN_POINT ( 'NONE',  ( -31.11269837220809364, -10.55634918610397932, 2.000000000000001776 ) ) ;
#43368=VECTOR ( 'NONE', #35885, 1000.000000000000000 ) ;
#43423=DIRECTION ( 'NONE',  ( 0.000000000000000000, 0.000000000000000000, 1.000000000000000000 ) ) ;
#43442=EDGE_CURVE ( 'NONE', #60938, #67479, #52902, .T. ) ;
#43447=ORIENTED_EDGE ( 'NONE', *, *, #67362, .T. ) ;
#43449=DIRECTION ( 'NONE',  ( 0.000000000000000000, 0.000000000000000000, 1.000000000000000000 ) ) ;
#43454=EDGE_LOOP ( 'NONE', ( #31530, #54291, #39496, #55035 ) ) ;
#43462=AXIS2_PLACEMENT_3D ( 'NONE', #4494, #42465, #37528 ) ;
#43465=PLANE ( 'NONE',  #34754 ) ;
#43468=ORIENTED_EDGE ( 'NONE', *, *, #36922, .T. ) ;
#43474=AXIS2_PLACEMENT_3D ( 'NONE', #59282, #27272, #26935 ) ;
#43495=LINE ( 'NONE', #64972, #11300 ) ;
#43516=VECTOR ( 'NONE', #21383, 1000.000000000000000 ) ;
#43522=CARTESIAN_POINT ( 'NONE',  ( 46.66904755831207297, -10.55634918610412853, 85.00100000000000477 ) ) ;
#43550=PLANE ( 'NONE',  #3636 ) ;
#43566=LINE ( 'NONE', #33390, #62230 ) ;
#43568=ORIENTED_EDGE ( 'NONE', *, *, #44854, .F. ) ;
#43578=AXIS2_PLACEMENT_3D ( 'NONE', #62437, #8974, #14252 ) ;
#43608=CARTESIAN_POINT ( 'NONE',  ( -36.11269837220812207, -31.11269837220801193, 0.000000000000000000 ) ) ;
#43617=CARTESIAN_POINT ( 'NONE',  ( 46.66904755831210139, -9.150666335777657423E-14, 85.00100000000000477 ) ) ;
#43619=ORIENTED_EDGE ( 'NONE', *, *, #46085, .F. ) ;
#43621=DIRECTION ( 'NONE',  ( 0.000000000000000000, 0.000000000000000000, 1.000000000000000000 ) ) ;
#43687=DIRECTION ( 'NONE',  ( -0.000000000000000000, -0.000000000000000000, 1.000000000000000000 ) ) ;
#43731=VERTEX_POINT ( 'NONE', #46868 ) ;
#43733=( NAMED_UNIT ( * ) PLANE_ANGLE_UNIT ( ) SI_UNIT ( $, .RADIAN. ) );
#43741=ORIENTED_EDGE ( 'NONE', *, *, #1826, .T. ) ;
#43742=ORIENTED_EDGE ( 'NONE', *, *, #59241, .T. ) ;
#43778=ORIENTED_EDGE ( 'NONE', *, *, #56361, .T. ) ;
#43802=CARTESIAN_POINT ( 'NONE',  ( 10.55634918610396511, -46.66904755831214402, 85.00100000000000477 ) ) ;
#43805=EDGE_CURVE ( 'NONE', #43873, #10912, #28888, .T. ) ;
#43813=VERTEX_POINT ( 'NONE', #13996 ) ;
#43818=CARTESIAN_POINT ( 'NONE',  ( -20.55634918610405748, -10.55634918610400597, 85.00100000000000477 ) ) ;
#43834=CARTESIAN_POINT ( 'NONE',  ( -20.55634918610408945, -31.11269837220804035, 2.000000000000000000 ) ) ;
#43838=EDGE_CURVE ( 'NONE', #32720, #58547, #51635, .T. ) ;
#43844=DIRECTION ( 'NONE',  ( 0.000000000000000000, -1.000000000000000000, 0.000000000000000000 ) ) ;
#43849=DIRECTION ( 'NONE',  ( 0.000000000000000000, 1.000000000000000000, 0.000000000000000000 ) ) ;
#43851=ORIENTED_EDGE ( 'NONE', *, *, #47153, .F. ) ;
#43854=DIRECTION ( 'NONE',  ( -0.000000000000000000, -0.000000000000000000, -1.000000000000000000 ) ) ;
#43872=PLANE ( 'NONE',  #11459 ) ;
#43873=VERTEX_POINT ( 'NONE', #1451 ) ;
#43890=CARTESIAN_POINT ( 'NONE',  ( 0.000000000000000000, 0.000000000000000000, 25.70156211871649887 ) ) ;
#43895=EDGE_CURVE ( 'NONE', #30095, #62805, #58617, .T. ) ;
#43917=CARTESIAN_POINT ( 'NONE',  ( 15.55634918610400241, -10.55634918610406281, 2.000000000000001776 ) ) ;
#43925=ORIENTED_EDGE ( 'NONE', *, *, #52485, .F. ) ;
#43926=DIRECTION ( 'NONE',  ( 1.000000000000000000, 0.000000000000000000, 0.000000000000000000 ) ) ;
#43936=DIRECTION ( 'NONE',  ( -0.000000000000000000, -0.000000000000000000, -1.000000000000000000 ) ) ;
#43937=CARTESIAN_POINT ( 'NONE',  ( -46.66904755831210139, 6.635317295611287136E-14, 0.000000000000000000 ) ) ;
#43938=AXIS2_PLACEMENT_3D ( 'NONE', #61786, #13608, #62135 ) ;
#43946=ORIENTED_EDGE ( 'NONE', *, *, #26432, .F. ) ;
#43954=CARTESIAN_POINT ( 'NONE',  ( 26.11269837220809364, 15.55634918610396866, 2.000000000000000000 ) ) ;
#43955=COLOUR_RGB ( '',0.7921568627450980005, 0.8196078431372548767, 0.9333333333333333481 ) ;
#43970=LINE ( 'NONE', #65452, #31207 ) ;
#44017=CARTESIAN_POINT ( 'NONE',  ( 15.55634918610397399, -26.11269837220809364, 0.000000000000000000 ) ) ;
#44029=ORIENTED_EDGE ( 'NONE', *, *, #790, .F. ) ;
#44061=DIRECTION ( 'NONE',  ( -0.000000000000000000, -0.000000000000000000, -1.000000000000000000 ) ) ;
#44102=CARTESIAN_POINT ( 'NONE',  ( -4.999999999999936939, 31.11269837220806167, 2.000000000000000000 ) ) ;
#44126=CARTESIAN_POINT ( 'NONE',  ( 31.11269837220809364, 15.55634918610396866, 0.000000000000000000 ) ) ;
#44130=DIRECTION ( 'NONE',  ( -1.000000000000000000, 0.000000000000000000, 0.000000000000000000 ) ) ;
#44142=PLANE ( 'NONE',  #17881 ) ;
#44161=CARTESIAN_POINT ( 'NONE',  ( -2.645453300864630819E-14, -15.55634918610403616, 0.000000000000000000 ) ) ;
#44196=VECTOR ( 'NONE', #35586, 1000.000000000000000 ) ;
#44205=CARTESIAN_POINT ( 'NONE',  ( -31.11269837220812207, -31.11269837220801193, 2.000000000000001776 ) ) ;
#44209=DIRECTION ( 'NONE',  ( -0.000000000000000000, -0.000000000000000000, -1.000000000000000000 ) ) ;
#44250=VERTEX_POINT ( 'NONE', #45027 ) ;
#44280=DIRECTION ( 'NONE',  ( 0.000000000000000000, 0.000000000000000000, 1.000000000000000000 ) ) ;
#44283=CARTESIAN_POINT ( 'NONE',  ( -36.11269837220806522, 5.000000000000056843, 2.000000000000001776 ) ) ;
#44284=EDGE_CURVE ( 'NONE', #12932, #38551, #1790, .T. ) ;
#44299=CARTESIAN_POINT ( 'NONE',  ( 46.66904755831210139, -9.150666335777657423E-14, 85.00100000000000477 ) ) ;
#44304=ORIENTED_EDGE ( 'NONE', *, *, #69086, .F. ) ;
#44305=ADVANCED_FACE ( 'NONE', ( #24636 ), #30252, .F. ) ;
#44311=CARTESIAN_POINT ( 'NONE',  ( 46.66904755831207297, -15.55634918610412853, 2.000000000000001776 ) ) ;
#44316=EDGE_LOOP ( 'NONE', ( #57835, #50783, #47012, #37460 ) ) ;
#44320=DIRECTION ( 'NONE',  ( -0.000000000000000000, -0.000000000000000000, -1.000000000000000000 ) ) ;
#44322=CARTESIAN_POINT ( 'NONE',  ( 10.55634918610411432, 46.66904755831205875, 85.00100000000000477 ) ) ;
#44330=FACE_OUTER_BOUND ( 'NONE', #50206, .T. ) ;
#44334=DIRECTION ( 'NONE',  ( -0.000000000000000000, -0.000000000000000000, -1.000000000000000000 ) ) ;
#44354=ORIENTED_EDGE ( 'NONE', *, *, #65252, .T. ) ;
#44358=CARTESIAN_POINT ( 'NONE',  ( -73.43826238111391547, 8.993593295997464589E-15, 26.24939009510892518 ) ) ;
#44405=VECTOR ( 'NONE', #31132, 1000.000000000000000 ) ;
#44411=ORIENTED_EDGE ( 'NONE', *, *, #59142, .T. ) ;
#44456=VECTOR ( 'NONE', #63466, 999.9999999999998863 ) ;
#44495=CARTESIAN_POINT ( 'NONE',  ( -15.55634918610408945, -26.11269837220804035, 2.000000000000001776 ) ) ;
#44498=VECTOR ( 'NONE', #54031, 1000.000000000000000 ) ;
#44510=DIRECTION ( 'NONE',  ( 0.000000000000000000, 1.000000000000000000, -0.000000000000000000 ) ) ;
#44556=PLANE ( 'NONE',  #37911 ) ;
#44558=DIRECTION ( 'NONE',  ( 0.000000000000000000, 0.000000000000000000, 1.000000000000000000 ) ) ;
#44561=DIRECTION ( 'NONE',  ( -0.000000000000000000, -1.000000000000000000, -0.000000000000000000 ) ) ;
#44568=EDGE_LOOP ( 'NONE', ( #26384, #48288, #21461, #27256 ) ) ;
#44584=CARTESIAN_POINT ( 'NONE',  ( 31.11269837220809364, 20.55634918610396866, 85.00100000000000477 ) ) ;
#44589=VERTEX_POINT ( 'NONE', #9833 ) ;
#44591=VECTOR ( 'NONE', #1459, 1000.000000000000000 ) ;
#44593=CARTESIAN_POINT ( 'NONE',  ( 15.55634918610406103, 20.55634918610400064, 2.000000000000001776 ) ) ;
#44599=AXIS2_PLACEMENT_3D ( 'NONE', #59975, #44510, #43449 ) ;
#44625=ORIENTED_EDGE ( 'NONE', *, *, #46516, .T. ) ;
#44669=ORIENTED_EDGE ( 'NONE', *, *, #38594, .F. ) ;
#44686=CARTESIAN_POINT ( 'NONE',  ( 31.11269837220806522, 4.999999999999936939, 0.000000000000000000 ) ) ;
#44707=FACE_OUTER_BOUND ( 'NONE', #55149, .T. ) ;
#44724=DIRECTION ( 'NONE',  ( -1.000000000000000000, 0.000000000000000000, 0.000000000000000000 ) ) ;
#44732=DIRECTION ( 'NONE',  ( 0.000000000000000000, 1.000000000000000000, 0.000000000000000000 ) ) ;
#44752=FACE_OUTER_BOUND ( 'NONE', #29966, .T. ) ;
#44757=LINE ( 'NONE', #27874, #49044 ) ;
#44758=AXIS2_PLACEMENT_3D ( 'NONE', #53759, #661, #22111 ) ;
#44786=EDGE_LOOP ( 'NONE', ( #19849, #45671, #13753, #50488 ) ) ;
#44792=EDGE_CURVE ( 'NONE', #17510, #56697, #40290, .T. ) ;
#44813=VERTEX_POINT ( 'NONE', #67042 ) ;
#44832=ORIENTED_EDGE ( 'NONE', *, *, #31868, .F. ) ;
#44834=LINE ( 'NONE', #23036, #39746 ) ;
#44840=ORIENTED_EDGE ( 'NONE', *, *, #62074, .T. ) ;
#44842=PLANE ( 'NONE',  #465 ) ;
#44850=CARTESIAN_POINT ( 'NONE',  ( -5.000000000000026645, -10.55634918610403439, 0.000000000000000000 ) ) ;
#44854=EDGE_CURVE ( 'NONE', #60938, #49516, #4041, .T. ) ;
#44880=ADVANCED_FACE ( 'NONE', ( #36744 ), #58187, .F. ) ;
#44916=CARTESIAN_POINT ( 'NONE',  ( 31.11269837220800127, -26.11269837220812562, 85.00100000000000477 ) ) ;
#44920=CARTESIAN_POINT ( 'NONE',  ( -31.11269837220801193, 36.11269837220812207, 85.00100000000000477 ) ) ;
#44939=DIRECTION ( 'NONE',  ( 1.000000000000000000, -0.000000000000000000, 0.000000000000000000 ) ) ;
#44956=ORIENTED_EDGE ( 'NONE', *, *, #31692, .F. ) ;
#44963=DIRECTION ( 'NONE',  ( -0.000000000000000000, -0.000000000000000000, -1.000000000000000000 ) ) ;
#44965=ORIENTED_EDGE ( 'NONE', *, *, #19182, .T. ) ;
#44982=ORIENTED_EDGE ( 'NONE', *, *, #61497, .F. ) ;
#44987=CARTESIAN_POINT ( 'NONE',  ( -5.000000000000058620, -31.11269837220806878, 85.00100000000000477 ) ) ;
#44999=CARTESIAN_POINT ( 'NONE',  ( 46.66904755831210139, 4.999999999999909406, 2.000000000000001776 ) ) ;
#45007=AXIS2_PLACEMENT_3D ( 'NONE', #48485, #59063, #16506 ) ;
#45027=CARTESIAN_POINT ( 'NONE',  ( -31.11269837220809364, -15.55634918610397754, 0.000000000000000000 ) ) ;
#45032=EDGE_CURVE ( 'NONE', #23803, #56265, #59553, .T. ) ;
#45042=FACE_OUTER_BOUND ( 'NONE', #23496, .T. ) ;
#45051=ORIENTED_EDGE ( 'NONE', *, *, #64616, .F. ) ;
#45064=DIRECTION ( 'NONE',  ( 0.000000000000000000, 0.000000000000000000, -1.000000000000000000 ) ) ;
#45072=LINE ( 'NONE', #33837, #53232 ) ;
#45081=EDGE_CURVE ( 'NONE', #27081, #39681, #1178, .T. ) ;
#45085=DIRECTION ( 'NONE',  ( 0.6246950475544236214, 0.000000000000000000, 0.7808688094430308313 ) ) ;
#45102=VECTOR ( 'NONE', #15845, 1000.000000000000000 ) ;
#45122=ORIENTED_EDGE ( 'NONE', *, *, #66157, .F. ) ;
#45145=ORIENTED_EDGE ( 'NONE', *, *, #56996, .F. ) ;
#45167=VECTOR ( 'NONE', #50496, 1000.000000000000000 ) ;
#45169=EDGE_CURVE ( 'NONE', #54143, #34238, #33893, .T. ) ;
#45172=EDGE_LOOP ( 'NONE', ( #56479, #38756, #49867, #34213 ) ) ;
#45188=EDGE_CURVE ( 'NONE', #26154, #14102, #19785, .T. ) ;
#45236=DIRECTION ( 'NONE',  ( -0.000000000000000000, -0.000000000000000000, -1.000000000000000000 ) ) ;
#45270=EDGE_LOOP ( 'NONE', ( #14854, #27529, #29511, #30391 ) ) ;
#45275=VECTOR ( 'NONE', #27644, 1000.000000000000000 ) ;
#45300=ORIENTED_EDGE ( 'NONE', *, *, #36703, .T. ) ;
#45312=VECTOR ( 'NONE', #54931, 1000.000000000000000 ) ;
#45335=DIRECTION ( 'NONE',  ( 0.000000000000000000, 1.000000000000000000, -0.000000000000000000 ) ) ;
#45341=APPLICATION_CONTEXT ( 'automotive_design' ) ;
#45352=CARTESIAN_POINT ( 'NONE',  ( 15.55634918610403261, -3.079134169858832593E-14, 2.000000000000001776 ) ) ;
#45389=ORIENTED_EDGE ( 'NONE', *, *, #20941, .F. ) ;
#45391=CARTESIAN_POINT ( 'NONE',  ( 46.66904755831207297, -15.55634918610412853, 2.000000000000001776 ) ) ;
#45408=DIRECTION ( 'NONE',  ( -0.6246950475544236214, 7.650307904307285654E-17, 0.7808688094430308313 ) ) ;
#45409=DIRECTION ( 'NONE',  ( 0.000000000000000000, 1.000000000000000000, -0.000000000000000000 ) ) ;
#45410=CARTESIAN_POINT ( 'NONE',  ( 15.55634918610396511, -41.66904755831214402, 2.000000000000001776 ) ) ;
#45426=VERTEX_POINT ( 'NONE', #4978 ) ;
#45434=EDGE_LOOP ( 'NONE', ( #18692, #34587, #8755, #8741 ) ) ;
#45435=DIRECTION ( 'NONE',  ( 1.000000000000000000, 0.000000000000000000, 0.000000000000000000 ) ) ;
#45437=CARTESIAN_POINT ( 'NONE',  ( -31.11269837220801193, 36.11269837220812207, 2.000000000000001776 ) ) ;
#45446=CARTESIAN_POINT ( 'NONE',  ( -5.767955557622883589E-14, -26.11269837220806522, 2.000000000000001776 ) ) ;
#45450=LINE ( 'NONE', #66242, #36629 ) ;
#45462=VECTOR ( 'NONE', #58247, 1000.000000000000000 ) ;
#45464=CARTESIAN_POINT ( 'NONE',  ( 46.66904755831212981, 20.55634918610394379, 2.000000000000001776 ) ) ;
#45489=CARTESIAN_POINT ( 'NONE',  ( -31.11269837220809364, -15.55634918610397754, 2.000000000000001776 ) ) ;
#45502=AXIS2_PLACEMENT_3D ( 'NONE', #28430, #24483, #25859 ) ;
#45506=CARTESIAN_POINT ( 'NONE',  ( 0.000000000000000000, 0.000000000000000000, 2.000000000000001776 ) ) ;
#45512=DIRECTION ( 'NONE',  ( 0.000000000000000000, -0.000000000000000000, -1.000000000000000000 ) ) ;
#45514=FACE_OUTER_BOUND ( 'NONE', #14903, .T. ) ;
#45538=DIRECTION ( 'NONE',  ( 0.000000000000000000, 0.000000000000000000, 1.000000000000000000 ) ) ;
#45579=EDGE_CURVE ( 'NONE', #56240, #18531, #8816, .T. ) ;
#45581=EDGE_CURVE ( 'NONE', #23252, #41022, #35542, .T. ) ;
#45588=LINE ( 'NONE', #61075, #31055 ) ;
#45589=EDGE_CURVE ( 'NONE', #38519, #55744, #19701, .T. ) ;
#45645=FACE_BOUND ( 'NONE', #53654, .T. ) ;
#45661=CIRCLE ( 'NONE', #16428, 74.99999999999998579 ) ;
#45671=ORIENTED_EDGE ( 'NONE', *, *, #64306, .T. ) ;
#45680=LINE ( 'NONE', #40392, #26628 ) ;
#45686=ORIENTED_EDGE ( 'NONE', *, *, #12645, .T. ) ;
#45687=DIRECTION ( 'NONE',  ( 0.000000000000000000, 1.000000000000000000, -0.000000000000000000 ) ) ;
#45725=FACE_BOUND ( 'NONE', #11507, .T. ) ;
#45747=VECTOR ( 'NONE', #22166, 1000.000000000000000 ) ;
#45759=EDGE_CURVE ( 'NONE', #58934, #42033, #59044, .T. ) ;
#45761=CIRCLE ( 'NONE', #64881, 54.03875030502680943 ) ;
#45771=ORIENTED_EDGE ( 'NONE', *, *, #39313, .T. ) ;
#45779=VERTEX_POINT ( 'NONE', #16489 ) ;
#45820=EDGE_LOOP ( 'NONE', ( #13855, #24925, #57925, #64 ) ) ;
#45853=DIRECTION ( 'NONE',  ( 0.000000000000000000, 0.000000000000000000, 1.000000000000000000 ) ) ;
#45873=CARTESIAN_POINT ( 'NONE',  ( -15.55634918610396866, 31.11269837220809009, 85.00100000000000477 ) ) ;
#45884=EDGE_LOOP ( 'NONE', ( #40965, #7864, #8951, #29122 ) ) ;
#45887=LINE ( 'NONE', #30398, #50475 ) ;
#45898=ADVANCED_FACE ( 'NONE', ( #38288 ), #24214, .F. ) ;
#45899=AXIS2_PLACEMENT_3D ( 'NONE', #32112, #437, #60228 ) ;
#45919=EDGE_LOOP ( 'NONE', ( #13267, #17540, #2502, #51118 ) ) ;
#45930=ORIENTED_EDGE ( 'NONE', *, *, #60873, .T. ) ;
#45943=LINE ( 'NONE', #56151, #8204 ) ;
#45949=VECTOR ( 'NONE', #23414, 1000.000000000000000 ) ;
#45962=ORIENTED_EDGE ( 'NONE', *, *, #30054, .F. ) ;
#45966=EDGE_CURVE ( 'NONE', #11222, #327, #36145, .T. ) ;
#45968=EDGE_LOOP ( 'NONE', ( #7450, #47033, #63469, #51852 ) ) ;
#45994=ORIENTED_EDGE ( 'NONE', *, *, #24778, .F. ) ;
#46013=CARTESIAN_POINT ( 'NONE',  ( -5.000000000000058620, -31.11269837220806878, 85.00100000000000477 ) ) ;
#46019=VECTOR ( 'NONE', #16212, 1000.000000000000000 ) ;
#46067=ORIENTED_EDGE ( 'NONE', *, *, #52804, .F. ) ;
#46078=ORIENTED_EDGE ( 'NONE', *, *, #65531, .T. ) ;
#46083=CARTESIAN_POINT ( 'NONE',  ( 31.11269837220812562, 36.11269837220800838, 2.000000000000001776 ) ) ;
#46085=EDGE_CURVE ( 'NONE', #39331, #5030, #52990, .T. ) ;
#46105=FACE_OUTER_BOUND ( 'NONE', #47723, .T. ) ;
#46135=EDGE_LOOP ( 'NONE', ( #38654, #26305 ) ) ;
#46148=ORIENTED_EDGE ( 'NONE', *, *, #26436, .T. ) ;
#46168=CARTESIAN_POINT ( 'NONE',  ( 15.55634918610411610, 51.66904755831205875, 85.00100000000000477 ) ) ;
#46186=DIRECTION ( 'NONE',  ( 0.000000000000000000, -0.000000000000000000, -1.000000000000000000 ) ) ;
#46189=DIRECTION ( 'NONE',  ( -1.000000000000000000, 0.000000000000000000, 0.000000000000000000 ) ) ;
#46214=LINE ( 'NONE', #67694, #3491 ) ;
#46232=ORIENTED_EDGE ( 'NONE', *, *, #33358, .F. ) ;
#46241=ORIENTED_EDGE ( 'NONE', *, *, #63993, .T. ) ;
#46258=VECTOR ( 'NONE', #66165, 1000.000000000000000 ) ;
#46265=ORIENTED_EDGE ( 'NONE', *, *, #15982, .T. ) ;
#46272=AXIS2_PLACEMENT_3D ( 'NONE', #20717, #68563, #68887 ) ;
#46292=DIRECTION ( 'NONE',  ( 0.000000000000000000, 0.000000000000000000, 1.000000000000000000 ) ) ;
#46320=VERTEX_POINT ( 'NONE', #46879 ) ;
#46323=CARTESIAN_POINT ( 'NONE',  ( 31.11269837220806522, 4.999999999999936939, 85.00100000000000477 ) ) ;
#46330=EDGE_LOOP ( 'NONE', ( #5945, #68139, #67100, #888 ) ) ;
#46335=CARTESIAN_POINT ( 'NONE',  ( 46.66904755831212981, 15.55634918610394379, 85.00100000000000477 ) ) ;
#46344=VERTEX_POINT ( 'NONE', #20481 ) ;
#46372=VERTEX_POINT ( 'NONE', #32082 ) ;
#46387=LINE ( 'NONE', #43522, #848 ) ;
#46392=ADVANCED_FACE ( 'NONE', ( #16589 ), #38045, .F. ) ;
#46393=EDGE_CURVE ( 'NONE', #50563, #12932, #48924, .T. ) ;
#46396=EDGE_LOOP ( 'NONE', ( #15159, #26397, #11233, #31490 ) ) ;
#46400=AXIS2_PLACEMENT_3D ( 'NONE', #578, #51806, #35974 ) ;
#46402=ORIENTED_EDGE ( 'NONE', *, *, #25350, .T. ) ;
#46416=DIRECTION ( 'NONE',  ( -1.000000000000000000, 0.000000000000000000, 0.000000000000000000 ) ) ;
#46441=PLANE ( 'NONE',  #51304 ) ;
#46452=PLANE ( 'NONE',  #53218 ) ;
#46475=ORIENTED_EDGE ( 'NONE', *, *, #1768, .F. ) ;
#46482=EDGE_LOOP ( 'NONE', ( #38114, #1738, #47833, #50721 ) ) ;
#46489=EDGE_LOOP ( 'NONE', ( #35161, #29781, #66566, #32926 ) ) ;
#46493=FACE_BOUND ( 'NONE', #61988, .T. ) ;
#46498=VECTOR ( 'NONE', #9001, 1000.000000000000000 ) ;
#46501=VECTOR ( 'NONE', #27149, 1000.000000000000000 ) ;
#46504=CARTESIAN_POINT ( 'NONE',  ( -31.11269837220806878, 5.000000000000056843, 85.00100000000000477 ) ) ;
#46505=DIRECTION ( 'NONE',  ( -0.000000000000000000, -0.000000000000000000, -1.000000000000000000 ) ) ;
#46516=EDGE_CURVE ( 'NONE', #60552, #53918, #22914, .T. ) ;
#46522=ORIENTED_EDGE ( 'NONE', *, *, #8977, .F. ) ;
#46533=EDGE_CURVE ( 'NONE', #18069, #21122, #51040, .T. ) ;
#46561=EDGE_CURVE ( 'NONE', #21979, #43731, #28541, .T. ) ;
#46566=VECTOR ( 'NONE', #53213, 1000.000000000000000 ) ;
#46586=ORIENTED_EDGE ( 'NONE', *, *, #10230, .T. ) ;
#46592=LINE ( 'NONE', #30088, #42888 ) ;
#46600=EDGE_LOOP ( 'NONE', ( #54914, #12204, #67980, #40630 ) ) ;
#46601=EDGE_LOOP ( 'NONE', ( #39473, #16835, #33351, #5117 ) ) ;
#46603=CIRCLE ( 'NONE', #45502, 74.99999999999998579 ) ;
#46608=AXIS2_PLACEMENT_3D ( 'NONE', #920, #20049, #15794 ) ;
#46617=ORIENTED_EDGE ( 'NONE', *, *, #52976, .F. ) ;
#46630=EDGE_LOOP ( 'NONE', ( #35265, #3006, #13227, #64368 ) ) ;
#46659=VECTOR ( 'NONE', #39317, 1000.000000000000000 ) ;
#46664=PLANE ( 'NONE',  #38443 ) ;
#46673=ORIENTED_EDGE ( 'NONE', *, *, #54127, .F. ) ;
#46675=DIRECTION ( 'NONE',  ( -1.000000000000000000, 0.000000000000000000, 0.000000000000000000 ) ) ;
#46686=LINE ( 'NONE', #67139, #2361 ) ;
#46712=AXIS2_PLACEMENT_3D ( 'NONE', #45873, #29694, #24433 ) ;
#46713=VERTEX_POINT ( 'NONE', #42874 ) ;
#46742=CARTESIAN_POINT ( 'NONE',  ( 0.000000000000000000, 0.000000000000000000, 0.000000000000000000 ) ) ;
#46755=DIRECTION ( 'NONE',  ( -0.000000000000000000, -0.000000000000000000, -1.000000000000000000 ) ) ;
#46757=AXIS2_PLACEMENT_3D ( 'NONE', #25805, #47235, #53881 ) ;
#46797=ORIENTED_EDGE ( 'NONE', *, *, #23109, .F. ) ;
#46809=ORIENTED_EDGE ( 'NONE', *, *, #13966, .F. ) ;
#46810=CARTESIAN_POINT ( 'NONE',  ( -5.000000000000000000, 5.000000000000000000, 2.000000000000001776 ) ) ;
#46816=LINE ( 'NONE', #68284, #20553 ) ;
#46864=LINE ( 'NONE', #64071, #68481 ) ;
#46868=CARTESIAN_POINT ( 'NONE',  ( 10.55634918610409656, 36.11269837220803680, 2.000000000000001776 ) ) ;
#46879=CARTESIAN_POINT ( 'NONE',  ( 65.00000000000000000, 0.000000000000000000, 85.00000000000000000 ) ) ;
#46904=VECTOR ( 'NONE', #61604, 1000.000000000000000 ) ;
#46911=CARTESIAN_POINT ( 'NONE',  ( 15.55634918610400241, -15.55634918610406103, 85.00100000000000477 ) ) ;
#46925=DIRECTION ( 'NONE',  ( -0.000000000000000000, -0.000000000000000000, -1.000000000000000000 ) ) ;
#46935=EDGE_CURVE ( 'NONE', #10376, #37117, #64824, .T. ) ;
#46964=EDGE_CURVE ( 'NONE', #56852, #51103, #64266, .T. ) ;
#46996=PLANE ( 'NONE',  #42631 ) ;
#47012=ORIENTED_EDGE ( 'NONE', *, *, #16520, .F. ) ;
#47033=ORIENTED_EDGE ( 'NONE', *, *, #10290, .T. ) ;
#47058=ORIENTED_EDGE ( 'NONE', *, *, #26379, .T. ) ;
#47087=EDGE_CURVE ( 'NONE', #19070, #38482, #6212, .T. ) ;
#47088=CARTESIAN_POINT ( 'NONE',  ( 15.55634918610411610, 46.66904755831205875, 2.000000000000001776 ) ) ;
#47118=CARTESIAN_POINT ( 'NONE',  ( 31.11269837220812562, 36.11269837220800838, 0.000000000000000000 ) ) ;
#47153=EDGE_CURVE ( 'NONE', #15461, #68402, #2344, .T. ) ;
#47170=VERTEX_POINT ( 'NONE', #43834 ) ;
#47176=VECTOR ( 'NONE', #60373, 1000.000000000000000 ) ;
#47181=ORIENTED_EDGE ( 'NONE', *, *, #11076, .T. ) ;
#47189=CARTESIAN_POINT ( 'NONE',  ( -15.55634918610400597, 15.55634918610405748, 2.000000000000001776 ) ) ;
#47209=CARTESIAN_POINT ( 'NONE',  ( -4.999999999999936939, 31.11269837220806167, 85.00100000000000477 ) ) ;
#47224=UNCERTAINTY_MEASURE_WITH_UNIT (LENGTH_MEASURE( 1.000000000000000082E-05 ), #27565, 'distance_accuracy_value', 'NONE');
#47233=CARTESIAN_POINT ( 'NONE',  ( -20.55634918610403261, 5.000000000000028422, 2.000000000000001776 ) ) ;
#47235=DIRECTION ( 'NONE',  ( 1.000000000000000000, 0.000000000000000000, 0.000000000000000000 ) ) ;
#47237=EDGE_CURVE ( 'NONE', #64405, #60938, #62464, .T. ) ;
#47246=DIRECTION ( 'NONE',  ( 0.000000000000000000, -1.000000000000000000, 0.000000000000000000 ) ) ;
#47261=EDGE_CURVE ( 'NONE', #47170, #65715, #30451, .T. ) ;
#47295=VERTEX_POINT ( 'NONE', #23967 ) ;
#47299=PLANE ( 'NONE',  #48985 ) ;
#47300=VECTOR ( 'NONE', #55911, 1000.000000000000000 ) ;
#47316=EDGE_CURVE ( 'NONE', #64960, #17852, #55984, .T. ) ;
#47322=CARTESIAN_POINT ( 'NONE',  ( 31.11269837220809364, 20.55634918610396866, 85.00100000000000477 ) ) ;
#47326=ORIENTED_EDGE ( 'NONE', *, *, #23109, .T. ) ;
#47335=EDGE_CURVE ( 'NONE', #30237, #14714, #2175, .T. ) ;
#47340=EDGE_CURVE ( 'NONE', #15785, #59242, #55624, .T. ) ;
#47342=DIRECTION ( 'NONE',  ( -1.000000000000000000, 0.000000000000000000, 0.000000000000000000 ) ) ;
#47362=EDGE_LOOP ( 'NONE', ( #25920, #14659, #19740, #5255 ) ) ;
#47365=CARTESIAN_POINT ( 'NONE',  ( -36.11269837220812207, -31.11269837220801193, 0.000000000000000000 ) ) ;
#47398=EDGE_CURVE ( 'NONE', #27081, #37153, #50698, .T. ) ;
#47400=ORIENTED_EDGE ( 'NONE', *, *, #66970, .T. ) ;
#47401=AXIS2_PLACEMENT_3D ( 'NONE', #69564, #31952, #63955 ) ;
#47409=VECTOR ( 'NONE', #33086, 1000.000000000000000 ) ;
#47413=VECTOR ( 'NONE', #45687, 1000.000000000000000 ) ;
#47417=CARTESIAN_POINT ( 'NONE',  ( 15.55634918610411610, 46.66904755831205875, 85.00100000000000477 ) ) ;
#47421=DIRECTION ( 'NONE',  ( 1.000000000000000000, -0.000000000000000000, -0.000000000000000000 ) ) ;
#47433=DIRECTION ( 'NONE',  ( -0.000000000000000000, -0.000000000000000000, -1.000000000000000000 ) ) ;
#47457=PLANE ( 'NONE',  #62445 ) ;
#47464=PLANE ( 'NONE',  #60844 ) ;
#47506=VECTOR ( 'NONE', #41968, 1000.000000000000000 ) ;
#47529=DIRECTION ( 'NONE',  ( -0.000000000000000000, -0.000000000000000000, -1.000000000000000000 ) ) ;
#47549=VECTOR ( 'NONE', #23793, 1000.000000000000000 ) ;
#47555=ORIENTED_EDGE ( 'NONE', *, *, #63993, .F. ) ;
#47590=ORIENTED_EDGE ( 'NONE', *, *, #25293, .T. ) ;
#47599=ADVANCED_FACE ( 'NONE', ( #26393 ), #44556, .F. ) ;
#47601=ORIENTED_EDGE ( 'NONE', *, *, #51926, .F. ) ;
#47639=ORIENTED_EDGE ( 'NONE', *, *, #40094, .T. ) ;
#47646=ADVANCED_FACE ( 'NONE', ( #36945 ), #31661, .F. ) ;
#47680=CARTESIAN_POINT ( 'NONE',  ( -36.11269837220812207, -31.11269837220801193, 2.000000000000000000 ) ) ;
#47687=EDGE_CURVE ( 'NONE', #4856, #58000, #64016, .T. ) ;
#47695=VERTEX_POINT ( 'NONE', #15493 ) ;
#47723=EDGE_LOOP ( 'NONE', ( #6414, #7216, #46475, #29176 ) ) ;
#47775=DIRECTION ( 'NONE',  ( 1.000000000000000000, -0.000000000000000000, -0.000000000000000000 ) ) ;
#47813=ORIENTED_EDGE ( 'NONE', *, *, #55020, .T. ) ;
#47831=DIRECTION ( 'NONE',  ( 0.000000000000000000, -1.000000000000000000, 0.000000000000000000 ) ) ;
#47833=ORIENTED_EDGE ( 'NONE', *, *, #56596, .F. ) ;
#47843=VERTEX_POINT ( 'NONE', #44102 ) ;
#47907=ORIENTED_EDGE ( 'NONE', *, *, #23350, .F. ) ;
#47913=PLANE ( 'NONE',  #26303 ) ;
#47959=ORIENTED_EDGE ( 'NONE', *, *, #25887, .F. ) ;
#47960=ORIENTED_EDGE ( 'NONE', *, *, #12819, .F. ) ;
#47966=CARTESIAN_POINT ( 'NONE',  ( -15.55634918610405748, -10.55634918610400597, 0.000000000000000000 ) ) ;
#47982=ORIENTED_EDGE ( 'NONE', *, *, #50509, .F. ) ;
#47995=VECTOR ( 'NONE', #54878, 1000.000000000000000 ) ;
#48001=CARTESIAN_POINT ( 'NONE',  ( 41.66904755831210849, 4.999999999999909406, 0.000000000000000000 ) ) ;
#48020=EDGE_LOOP ( 'NONE', ( #56530, #30770, #39152, #66687 ) ) ;
#48029=ORIENTED_EDGE ( 'NONE', *, *, #43442, .F. ) ;
#48033=FACE_BOUND ( 'NONE', #44568, .T. ) ;
#48042=ADVANCED_FACE ( 'NONE', ( #58142 ), #20498, .F. ) ;
#48044=VERTEX_POINT ( 'NONE', #9960 ) ;
#48070=LINE ( 'NONE', #54740, #15023 ) ;
#48073=LINE ( 'NONE', #27664, #62479 ) ;
#48083=CARTESIAN_POINT ( 'NONE',  ( -31.11269837220804035, 20.55634918610408945, 2.000000000000001776 ) ) ;
#48111=CARTESIAN_POINT ( 'NONE',  ( 15.55634918610409656, 36.11269837220803680, 2.000000000000001776 ) ) ;
#48123=ORIENTED_EDGE ( 'NONE', *, *, #56304, .F. ) ;
#48163=PLANE ( 'NONE',  #24086 ) ;
#48173=PLANE ( 'NONE',  #11407 ) ;
#48186=VECTOR ( 'NONE', #975, 1000.000000000000000 ) ;
#48187=ORIENTED_EDGE ( 'NONE', *, *, #24944, .F. ) ;
#48200=DIRECTION ( 'NONE',  ( -0.000000000000000000, -0.000000000000000000, -1.000000000000000000 ) ) ;
#48214=PLANE ( 'NONE',  #55918 ) ;
#48244=CIRCLE ( 'NONE', #26929, 66.50000000000000000 ) ;
#48245=CARTESIAN_POINT ( 'NONE',  ( 46.66904755831212981, 15.55634918610394379, 85.00100000000000477 ) ) ;
#48270=VERTEX_POINT ( 'NONE', #10897 ) ;
#48274=VERTEX_POINT ( 'NONE', #21126 ) ;
#48288=ORIENTED_EDGE ( 'NONE', *, *, #37323, .T. ) ;
#48293=LINE ( 'NONE', #21580, #25550 ) ;
#48322=ORIENTED_EDGE ( 'NONE', *, *, #37954, .F. ) ;
#48397=VECTOR ( 'NONE', #60427, 1000.000000000000000 ) ;
#48410=ORIENTED_EDGE ( 'NONE', *, *, #48803, .T. ) ;
#48427=EDGE_LOOP ( 'NONE', ( #39508, #56610, #16990, #13893 ) ) ;
#48455=EDGE_CURVE ( 'NONE', #5030, #36947, #55910, .T. ) ;
#48461=ORIENTED_EDGE ( 'NONE', *, *, #26581, .F. ) ;
#48469=EDGE_CURVE ( 'NONE', #25366, #18610, #38681, .T. ) ;
#48470=CARTESIAN_POINT ( 'NONE',  ( 7.762887554996211747E-14, 51.66904755831208718, 85.00100000000000477 ) ) ;
#48485=CARTESIAN_POINT ( 'NONE',  ( -46.66904755831210139, 6.635317295611287136E-14, 85.00100000000000477 ) ) ;
#48499=FACE_OUTER_BOUND ( 'NONE', #1381, .T. ) ;
#48502=ORIENTED_EDGE ( 'NONE', *, *, #34324, .T. ) ;
#48514=CARTESIAN_POINT ( 'NONE',  ( 15.55634918610409656, 36.11269837220803680, 2.000000000000001776 ) ) ;
#48520=DIRECTION ( 'NONE',  ( 0.000000000000000000, -0.000000000000000000, -1.000000000000000000 ) ) ;
#48544=DIRECTION ( 'NONE',  ( 0.000000000000000000, -1.000000000000000000, 0.000000000000000000 ) ) ;
#48547=ORIENTED_EDGE ( 'NONE', *, *, #24071, .F. ) ;
#48556=LINE ( 'NONE', #27469, #12342 ) ;
#48585=EDGE_CURVE ( 'NONE', #8745, #31701, #10474, .T. ) ;
#48603=CARTESIAN_POINT ( 'NONE',  ( -5.000000000000026645, -15.55634918610403616, 0.000000000000000000 ) ) ;
#48604=DIRECTION ( 'NONE',  ( 1.000000000000000000, -0.000000000000000000, 0.000000000000000000 ) ) ;
#48610=ORIENTED_EDGE ( 'NONE', *, *, #2837, .T. ) ;
#48625=LINE ( 'NONE', #42683, #2224 ) ;
#48647=DIRECTION ( 'NONE',  ( 0.000000000000000000, 1.000000000000000000, -0.000000000000000000 ) ) ;
#48662=ORIENTED_EDGE ( 'NONE', *, *, #61615, .F. ) ;
#48687=ORIENTED_EDGE ( 'NONE', *, *, #35697, .T. ) ;
#48688=VECTOR ( 'NONE', #45853, 1000.000000000000000 ) ;
#48715=CARTESIAN_POINT ( 'NONE',  ( -15.55634918610405748, -10.55634918610400597, 0.000000000000000000 ) ) ;
#48731=ORIENTED_EDGE ( 'NONE', *, *, #55592, .F. ) ;
#48737=FACE_OUTER_BOUND ( 'NONE', #23996, .T. ) ;
#48745=VECTOR ( 'NONE', #33401, 1000.000000000000000 ) ;
#48751=VERTEX_POINT ( 'NONE', #17484 ) ;
#48763=LINE ( 'NONE', #16770, #65451 ) ;
#48803=EDGE_CURVE ( 'NONE', #62926, #47295, #23482, .T. ) ;
#48804=DIRECTION ( 'NONE',  ( -0.000000000000000000, -0.000000000000000000, 1.000000000000000000 ) ) ;
#48817=PLANE ( 'NONE',  #44758 ) ;
#48832=CARTESIAN_POINT ( 'NONE',  ( 10.55634918610403084, -3.079134169858832593E-14, 0.000000000000000000 ) ) ;
#48861=FACE_OUTER_BOUND ( 'NONE', #28965, .T. ) ;
#48886=VECTOR ( 'NONE', #59869, 1000.000000000000000 ) ;
#48894=DIRECTION ( 'NONE',  ( -1.000000000000000000, 0.000000000000000000, 0.000000000000000000 ) ) ;
#48898=ORIENTED_EDGE ( 'NONE', *, *, #38765, .F. ) ;
#48912=DIRECTION ( 'NONE',  ( 0.000000000000000000, 1.000000000000000000, -0.000000000000000000 ) ) ;
#48924=LINE ( 'NONE', #38392, #55848 ) ;
#48951=ORIENTED_EDGE ( 'NONE', *, *, #50004, .T. ) ;
#48965=EDGE_CURVE ( 'NONE', #50563, #24929, #11330, .T. ) ;
#48971=ADVANCED_FACE ( 'NONE', ( #27868 ), #27163, .F. ) ;
#48977=LINE ( 'NONE', #54251, #56421 ) ;
#48985=AXIS2_PLACEMENT_3D ( 'NONE', #15310, #4743, #52918 ) ;
#48987=ORIENTED_EDGE ( 'NONE', *, *, #58801, .F. ) ;
#48988=EDGE_LOOP ( 'NONE', ( #42623, #15441, #25195, #62839 ) ) ;
#48990=EDGE_CURVE ( 'NONE', #27835, #61270, #49307, .T. ) ;
#48999=DIRECTION ( 'NONE',  ( 0.000000000000000000, -1.000000000000000000, 0.000000000000000000 ) ) ;
#49000=CARTESIAN_POINT ( 'NONE',  ( 15.55634918610406103, 20.55634918610400064, 2.000000000000001776 ) ) ;
#49026=( LENGTH_UNIT ( ) NAMED_UNIT ( * ) SI_UNIT ( .MILLI., .METRE. ) );
#49034=ADVANCED_FACE ( 'NONE', ( #26831 ), #38070, .F. ) ;
#49039=CARTESIAN_POINT ( 'NONE',  ( 0.000000000000000000, 0.000000000000000000, 85.00000000000000000 ) ) ;
#49044=VECTOR ( 'NONE', #12046, 1000.000000000000000 ) ;
#49055=DIRECTION ( 'NONE',  ( 1.000000000000000000, -0.000000000000000000, 0.000000000000000000 ) ) ;
#49065=VERTEX_POINT ( 'NONE', #59170 ) ;
#49099=EDGE_LOOP ( 'NONE', ( #16544, #2161, #42116, #14323 ) ) ;
#49117=CARTESIAN_POINT ( 'NONE',  ( 41.66904755831208007, -10.55634918610412853, 2.000000000000001776 ) ) ;
#49131=LINE ( 'NONE', #13859, #12793 ) ;
#49145=DIRECTION ( 'NONE',  ( 0.000000000000000000, -0.000000000000000000, -1.000000000000000000 ) ) ;
#49171=DIRECTION ( 'NONE',  ( 0.000000000000000000, 0.000000000000000000, 1.000000000000000000 ) ) ;
#49182=ORIENTED_EDGE ( 'NONE', *, *, #26354, .F. ) ;
#49210=EDGE_CURVE ( 'NONE', #11106, #47843, #67265, .T. ) ;
#49219=CARTESIAN_POINT ( 'NONE',  ( 46.66904755831212981, 20.55634918610394379, 85.00100000000000477 ) ) ;
#49222=LINE ( 'NONE', #34119, #41394 ) ;
#49251=DIRECTION ( 'NONE',  ( -0.000000000000000000, -0.000000000000000000, -1.000000000000000000 ) ) ;
#49259=DIRECTION ( 'NONE',  ( 1.000000000000000000, 0.000000000000000000, 0.000000000000000000 ) ) ;
#49295=EDGE_LOOP ( 'NONE', ( #47907, #120, #69169, #20101 ) ) ;
#49306=EDGE_LOOP ( 'NONE', ( #21447, #10578, #17951, #28663 ) ) ;
#49307=LINE ( 'NONE', #65513, #60456 ) ;
#49313=ADVANCED_FACE ( 'NONE', ( #44752 ), #23988, .F. ) ;
#49315=EDGE_LOOP ( 'NONE', ( #31468, #17581, #62300, #13667 ) ) ;
#49319=EDGE_LOOP ( 'NONE', ( #27387, #45300, #15206, #22072 ) ) ;
#49336=AXIS2_PLACEMENT_3D ( 'NONE', #20521, #31102, #25824 ) ;
#49338=DIRECTION ( 'NONE',  ( 0.000000000000000000, 0.000000000000000000, 1.000000000000000000 ) ) ;
#49366=ORIENTED_EDGE ( 'NONE', *, *, #36875, .F. ) ;
#49399=EDGE_CURVE ( 'NONE', #15169, #5346, #63700, .T. ) ;
#49405=ORIENTED_EDGE ( 'NONE', *, *, #20253, .F. ) ;
#49410=ORIENTED_EDGE ( 'NONE', *, *, #28764, .F. ) ;
#49418=ORIENTED_EDGE ( 'NONE', *, *, #55857, .F. ) ;
#49420=FACE_BOUND ( 'NONE', #30242, .T. ) ;
#49456=DIRECTION ( 'NONE',  ( 0.000000000000000000, -1.000000000000000000, 0.000000000000000000 ) ) ;
#49488=DIRECTION ( 'NONE',  ( -0.000000000000000000, -0.000000000000000000, -1.000000000000000000 ) ) ;
#49516=VERTEX_POINT ( 'NONE', #33430 ) ;
#49553=CARTESIAN_POINT ( 'NONE',  ( -20.55634918610400419, 15.55634918610405748, 2.000000000000001776 ) ) ;
#49557=CARTESIAN_POINT ( 'NONE',  ( 15.55634918610397399, -31.11269837220809364, 85.00100000000000477 ) ) ;
#49560=LINE ( 'NONE', #7021, #1271 ) ;
#49569=FACE_OUTER_BOUND ( 'NONE', #10859, .T. ) ;
#49577=CARTESIAN_POINT ( 'NONE',  ( -15.55634918610396866, 31.11269837220809009, 85.00100000000000477 ) ) ;
#49589=EDGE_CURVE ( 'NONE', #42920, #1235, #64370, .T. ) ;
#49590=DIRECTION ( 'NONE',  ( 0.000000000000000000, 0.000000000000000000, 1.000000000000000000 ) ) ;
#49599=CARTESIAN_POINT ( 'NONE',  ( -36.11269837220806522, 5.594483210025202879E-14, 0.000000000000000000 ) ) ;
#49610=AXIS2_PLACEMENT_3D ( 'NONE', #60146, #33437, #54863 ) ;
#49612=DIRECTION ( 'NONE',  ( 0.000000000000000000, 1.000000000000000000, -0.000000000000000000 ) ) ;
#49621=EDGE_LOOP ( 'NONE', ( #17285, #27886, #18422, #28387 ) ) ;
#49644=ORIENTED_EDGE ( 'NONE', *, *, #63127, .F. ) ;
#49669=CARTESIAN_POINT ( 'NONE',  ( -15.55634918610405748, -10.55634918610400597, 85.00100000000000477 ) ) ;
#49687=FACE_OUTER_BOUND ( 'NONE', #47362, .T. ) ;
#49700=ORIENTED_EDGE ( 'NONE', *, *, #62105, .T. ) ;
#49702=ORIENTED_EDGE ( 'NONE', *, *, #39700, .F. ) ;
#49705=DIRECTION ( 'NONE',  ( -0.000000000000000000, -0.000000000000000000, -1.000000000000000000 ) ) ;
#49712=LINE ( 'NONE', #17363, #25862 ) ;
#49744=EDGE_LOOP ( 'NONE', ( #44354, #44625, #60263, #43468 ) ) ;
#49751=LINE ( 'NONE', #66664, #49870 ) ;
#49767=EDGE_CURVE ( 'NONE', #40273, #57137, #63618, .T. ) ;
#49791=EDGE_CURVE ( 'NONE', #3346, #46713, #46387, .T. ) ;
#49793=LINE ( 'NONE', #1620, #21695 ) ;
#49794=CARTESIAN_POINT ( 'NONE',  ( 6.375108774214766072E-14, 31.11269837220806167, 2.000000000000001776 ) ) ;
#49798=EDGE_CURVE ( 'NONE', #23417, #67479, #16107, .T. ) ;
#49803=LINE ( 'NONE', #28718, #38538 ) ;
#49814=AXIS2_PLACEMENT_3D ( 'NONE', #12978, #40729, #34084 ) ;
#49824=LINE ( 'NONE', #23110, #34384 ) ;
#49830=LINE ( 'NONE', #12921, #30715 ) ;
#49839=EDGE_CURVE ( 'NONE', #62781, #17818, #26330, .T. ) ;
#49847=LINE ( 'NONE', #6951, #46659 ) ;
#49858=EDGE_CURVE ( 'NONE', #64201, #26921, #64652, .T. ) ;
#49866=VECTOR ( 'NONE', #45236, 1000.000000000000000 ) ;
#49867=ORIENTED_EDGE ( 'NONE', *, *, #42450, .F. ) ;
#49870=VECTOR ( 'NONE', #50470, 1000.000000000000000 ) ;
#49873=VECTOR ( 'NONE', #21643, 1000.000000000000000 ) ;
#49878=ORIENTED_EDGE ( 'NONE', *, *, #45589, .T. ) ;
#49879=VECTOR ( 'NONE', #33140, 1000.000000000000000 ) ;
#49887=EDGE_CURVE ( 'NONE', #65236, #30808, #38252, .T. ) ;
#49907=PLANE ( 'NONE',  #7094 ) ;
#49924=LINE ( 'NONE', #55916, #62782 ) ;
#49933=PLANE ( 'NONE',  #11441 ) ;
#49952=CARTESIAN_POINT ( 'NONE',  ( 65.00000000000000000, 0.000000000000000000, -0.002000000000002000178 ) ) ;
#49986=LINE ( 'NONE', #60544, #18343 ) ;
#49994=EDGE_LOOP ( 'NONE', ( #67696, #23324, #65076, #9910 ) ) ;
#49996=PLANE ( 'NONE',  #2886 ) ;
#50004=EDGE_CURVE ( 'NONE', #19565, #38069, #38607, .T. ) ;
#50025=VECTOR ( 'NONE', #67248, 1000.000000000000000 ) ;
#50036=CARTESIAN_POINT ( 'NONE',  ( 10.55634918610411432, 46.66904755831205875, 0.000000000000000000 ) ) ;
#50053=CARTESIAN_POINT ( 'NONE',  ( -5.767955557622883589E-14, -26.11269837220806522, 85.00100000000000477 ) ) ;
#50085=ORIENTED_EDGE ( 'NONE', *, *, #48990, .T. ) ;
#50102=CARTESIAN_POINT ( 'NONE',  ( 2.905661822261151883E-14, 20.55634918610402906, 85.00100000000000477 ) ) ;
#50109=DIRECTION ( 'NONE',  ( -1.000000000000000000, 0.000000000000000000, 0.000000000000000000 ) ) ;
#50122=FACE_OUTER_BOUND ( 'NONE', #41014, .T. ) ;
#50137=ORIENTED_EDGE ( 'NONE', *, *, #22704, .F. ) ;
#50145=ORIENTED_EDGE ( 'NONE', *, *, #39019, .T. ) ;
#50158=CARTESIAN_POINT ( 'NONE',  ( -36.11269837220806522, 5.594483210025202879E-14, 0.000000000000000000 ) ) ;
#50161=EDGE_CURVE ( 'NONE', #23252, #56240, #32896, .T. ) ;
#50168=ORIENTED_EDGE ( 'NONE', *, *, #50642, .F. ) ;
#50175=VECTOR ( 'NONE', #26392, 1000.000000000000000 ) ;
#50190=VECTOR ( 'NONE', #1344, 1000.000000000000000 ) ;
#50206=EDGE_LOOP ( 'NONE', ( #51182, #15438, #11490, #58461 ) ) ;
#50226=LINE ( 'NONE', #23501, #35314 ) ;
#50237=CARTESIAN_POINT ( 'NONE',  ( 54.03875030502680943, 0.000000000000000000, 2.000000000000001776 ) ) ;
#50262=CARTESIAN_POINT ( 'NONE',  ( -36.11269837220801548, 31.11269837220812207, 85.00100000000000477 ) ) ;
#50277=VECTOR ( 'NONE', #34543, 1000.000000000000000 ) ;
#50283=CARTESIAN_POINT ( 'NONE',  ( 41.66904755831208007, -10.55634918610412853, 0.000000000000000000 ) ) ;
#50288=CARTESIAN_POINT ( 'NONE',  ( 10.55634918610397577, -31.11269837220809364, 0.000000000000000000 ) ) ;
#50294=ORIENTED_EDGE ( 'NONE', *, *, #65858, .T. ) ;
#50309=ORIENTED_EDGE ( 'NONE', *, *, #53757, .T. ) ;
#50324=ORIENTED_EDGE ( 'NONE', *, *, #11098, .F. ) ;
#50340=CARTESIAN_POINT ( 'NONE',  ( -20.55634918610405748, -15.55634918610400774, 0.000000000000000000 ) ) ;
#50341=EDGE_LOOP ( 'NONE', ( #2538, #57643, #8886, #6253 ) ) ;
#50345=ORIENTED_EDGE ( 'NONE', *, *, #4327, .T. ) ;
#50357=CARTESIAN_POINT ( 'NONE',  ( -15.55634918610405748, -15.55634918610400774, 2.000000000000001776 ) ) ;
#50363=EDGE_CURVE ( 'NONE', #192, #19283, #50816, .T. ) ;
#50379=CARTESIAN_POINT ( 'NONE',  ( 15.55634918610403261, 4.999999999999969802, 85.00100000000000477 ) ) ;
#50413=CARTESIAN_POINT ( 'NONE',  ( -74.99999999999998579, 0.000000000000000000, 25.00000000000007816 ) ) ;
#50422=ADVANCED_FACE ( 'NONE', ( #35691 ), #8952, .F. ) ;
#50424=VERTEX_POINT ( 'NONE', #24098 ) ;
#50454=LINE ( 'NONE', #50102, #21710 ) ;
#50470=DIRECTION ( 'NONE',  ( 0.000000000000000000, 1.000000000000000000, -0.000000000000000000 ) ) ;
#50475=VECTOR ( 'NONE', #14227, 1000.000000000000000 ) ;
#50488=ORIENTED_EDGE ( 'NONE', *, *, #40094, .F. ) ;
#50496=DIRECTION ( 'NONE',  ( -0.000000000000000000, -0.000000000000000000, -1.000000000000000000 ) ) ;
#50509=EDGE_CURVE ( 'NONE', #16366, #44589, #66423, .T. ) ;
#50530=CARTESIAN_POINT ( 'NONE',  ( 0.000000000000000000, 0.000000000000000000, 0.000000000000000000 ) ) ;
#50533=FACE_OUTER_BOUND ( 'NONE', #58918, .T. ) ;
#50563=VERTEX_POINT ( 'NONE', #28409 ) ;
#50604=EDGE_CURVE ( 'NONE', #6738, #17255, #11180, .T. ) ;
#50609=VERTEX_POINT ( 'NONE', #59370 ) ;
#50610=DIRECTION ( 'NONE',  ( -0.000000000000000000, -0.000000000000000000, -1.000000000000000000 ) ) ;
#50641=ORIENTED_EDGE ( 'NONE', *, *, #38769, .F. ) ;
#50642=EDGE_CURVE ( 'NONE', #15785, #37709, #28059, .T. ) ;
#50648=VECTOR ( 'NONE', #31377, 1000.000000000000000 ) ;
#50654=EDGE_CURVE ( 'NONE', #26077, #58934, #22789, .T. ) ;
#50669=LINE ( 'NONE', #13393, #8862 ) ;
#50698=LINE ( 'NONE', #66552, #31198 ) ;
#50704=ORIENTED_EDGE ( 'NONE', *, *, #64790, .F. ) ;
#50721=ORIENTED_EDGE ( 'NONE', *, *, #10872, .F. ) ;
#50738=AXIS2_PLACEMENT_3D ( 'NONE', #27038, #60088, #1361 ) ;
#50747=ORIENTED_EDGE ( 'NONE', *, *, #3482, .F. ) ;
#50750=VERTEX_POINT ( 'NONE', #4457 ) ;
#50762=ORIENTED_EDGE ( 'NONE', *, *, #8977, .T. ) ;
#50765=FACE_OUTER_BOUND ( 'NONE', #22922, .T. ) ;
#50783=ORIENTED_EDGE ( 'NONE', *, *, #45966, .T. ) ;
#50807=EDGE_CURVE ( 'NONE', #10912, #51932, #59977, .T. ) ;
#50810=ORIENTED_EDGE ( 'NONE', *, *, #26764, .F. ) ;
#50816=LINE ( 'NONE', #67701, #39068 ) ;
#50892=DIRECTION ( 'NONE',  ( -0.000000000000000000, -0.000000000000000000, -1.000000000000000000 ) ) ;
#50922=ORIENTED_EDGE ( 'NONE', *, *, #63361, .F. ) ;
#50930=ORIENTED_EDGE ( 'NONE', *, *, #15247, .F. ) ;
#50936=VECTOR ( 'NONE', #40731, 1000.000000000000000 ) ;
#51040=LINE ( 'NONE', #7084, #44591 ) ;
#51067=CARTESIAN_POINT ( 'NONE',  ( 46.66904755831207297, -15.55634918610412853, 85.00100000000000477 ) ) ;
#51077=DIRECTION ( 'NONE',  ( 0.000000000000000000, 1.000000000000000000, -0.000000000000000000 ) ) ;
#51083=DIRECTION ( 'NONE',  ( 1.000000000000000000, -0.000000000000000000, -0.000000000000000000 ) ) ;
#51094=AXIS2_PLACEMENT_3D ( 'NONE', #25959, #5188, #5863 ) ;
#51095=VECTOR ( 'NONE', #19233, 1000.000000000000000 ) ;
#51103=VERTEX_POINT ( 'NONE', #6788 ) ;
#51110=DIRECTION ( 'NONE',  ( 0.000000000000000000, 0.000000000000000000, -1.000000000000000000 ) ) ;
#51118=ORIENTED_EDGE ( 'NONE', *, *, #55020, .F. ) ;
#51125=CARTESIAN_POINT ( 'NONE',  ( 15.55634918610409656, 31.11269837220803325, 0.000000000000000000 ) ) ;
#51126=EDGE_CURVE ( 'NONE', #49516, #13372, #32482, .T. ) ;
#51141=VECTOR ( 'NONE', #2188, 1000.000000000000000 ) ;
#51146=CARTESIAN_POINT ( 'NONE',  ( -51.66904755831210139, 5.000000000000066613, 2.000000000000001776 ) ) ;
#51149=( GEOMETRIC_REPRESENTATION_CONTEXT ( 3 ) GLOBAL_UNCERTAINTY_ASSIGNED_CONTEXT ( ( #23380 ) ) GLOBAL_UNIT_ASSIGNED_CONTEXT ( ( #49026, #4751, #32522 ) ) REPRESENTATION_CONTEXT ( 'NONE', 'WORKASPACE' ) );
#51157=VERTEX_POINT ( 'NONE', #45464 ) ;
#51168=LINE ( 'NONE', #57139, #61133 ) ;
#51169=FACE_OUTER_BOUND ( 'NONE', #55854, .T. ) ;
#51170=CARTESIAN_POINT ( 'NONE',  ( -36.11269837220812207, -26.11269837220801193, 85.00100000000000477 ) ) ;
#51176=EDGE_CURVE ( 'NONE', #17818, #54143, #66598, .T. ) ;
#51178=ADVANCED_FACE ( 'NONE', ( #8539 ), #28605, .F. ) ;
#51182=ORIENTED_EDGE ( 'NONE', *, *, #64790, .T. ) ;
#51192=VECTOR ( 'NONE', #42991, 1000.000000000000000 ) ;
#51223=CARTESIAN_POINT ( 'NONE',  ( 46.66904755831212981, 20.55634918610394379, 85.00100000000000477 ) ) ;
#51227=ORIENTED_EDGE ( 'NONE', *, *, #13459, .T. ) ;
#51255=CARTESIAN_POINT ( 'NONE',  ( -15.55634918610396866, 31.11269837220809009, 0.000000000000000000 ) ) ;
#51281=CARTESIAN_POINT ( 'NONE',  ( 15.55634918610403261, -3.079134169858832593E-14, 85.00100000000000477 ) ) ;
#51289=CARTESIAN_POINT ( 'NONE',  ( -4.999999999999971578, 15.55634918610403084, 0.000000000000000000 ) ) ;
#51295=LINE ( 'NONE', #6983, #61743 ) ;
#51299=EDGE_CURVE ( 'NONE', #37153, #10970, #54532, .T. ) ;
#51304=AXIS2_PLACEMENT_3D ( 'NONE', #67242, #25703, #24322 ) ;
#51338=CARTESIAN_POINT ( 'NONE',  ( 15.55634918610400241, -10.55634918610406281, 85.00100000000000477 ) ) ;
#51346=ORIENTED_EDGE ( 'NONE', *, *, #5092, .F. ) ;
#51347=CONICAL_SURFACE ( 'NONE', #29999, 74.99999999999998579, 0.6747409422235518539 ) ;
#51355=ORIENTED_EDGE ( 'NONE', *, *, #54278, .F. ) ;
#51362=CARTESIAN_POINT ( 'NONE',  ( 26.11269837220806167, -6.375108774214766072E-14, 85.00100000000000477 ) ) ;
#51363=CARTESIAN_POINT ( 'NONE',  ( 7.762887554996211747E-14, 46.66904755831208718, 0.000000000000000000 ) ) ;
#51380=EDGE_CURVE ( 'NONE', #53918, #3968, #16562, .T. ) ;
#51381=DIRECTION ( 'NONE',  ( 0.000000000000000000, 1.000000000000000000, -0.000000000000000000 ) ) ;
#51386=EDGE_CURVE ( 'NONE', #68402, #39331, #16214, .T. ) ;
#51390=AXIS2_PLACEMENT_3D ( 'NONE', #24417, #41616, #52171 ) ;
#51399=VECTOR ( 'NONE', #48894, 1000.000000000000000 ) ;
#51403=PLANE ( 'NONE',  #30956 ) ;
#51412=CARTESIAN_POINT ( 'NONE',  ( 0.000000000000000000, 0.000000000000000000, 2.000000000000001776 ) ) ;
#51441=AXIS2_PLACEMENT_3D ( 'NONE', #2998, #7227, #30412 ) ;
#51518=DIRECTION ( 'NONE',  ( -0.000000000000000000, -0.000000000000000000, -1.000000000000000000 ) ) ;
#51555=CARTESIAN_POINT ( 'NONE',  ( -36.11269837220806522, 5.000000000000056843, 0.000000000000000000 ) ) ;
#51561=ORIENTED_EDGE ( 'NONE', *, *, #49399, .F. ) ;
#51563=EDGE_LOOP ( 'NONE', ( #8574, #58300, #13980, #4358 ) ) ;
#51572=EDGE_CURVE ( 'NONE', #2018, #45426, #56988, .T. ) ;
#51603=DIRECTION ( 'NONE',  ( 0.000000000000000000, 1.000000000000000000, 0.000000000000000000 ) ) ;
#51604=CARTESIAN_POINT ( 'NONE',  ( 0.000000000000000000, 0.000000000000000000, 85.00000000000000000 ) ) ;
#51617=FACE_BOUND ( 'NONE', #26830, .T. ) ;
#51627=AXIS2_PLACEMENT_3D ( 'NONE', #51783, #40879, #3258 ) ;
#51635=LINE ( 'NONE', #6724, #64630 ) ;
#51672=VERTEX_POINT ( 'NONE', #68902 ) ;
#51679=DIRECTION ( 'NONE',  ( -0.000000000000000000, -0.000000000000000000, -1.000000000000000000 ) ) ;
#51685=ORIENTED_EDGE ( 'NONE', *, *, #60333, .F. ) ;
#51695=AXIS2_PLACEMENT_3D ( 'NONE', #59125, #27467, #22204 ) ;
#51698=ORIENTED_EDGE ( 'NONE', *, *, #48585, .F. ) ;
#51701=DIRECTION ( 'NONE',  ( -0.000000000000000000, -1.000000000000000000, -0.000000000000000000 ) ) ;
#51717=CARTESIAN_POINT ( 'NONE',  ( 10.55634918610406281, 15.55634918610400241, 0.000000000000000000 ) ) ;
#51722=ORIENTED_EDGE ( 'NONE', *, *, #48455, .F. ) ;
#51727=DIRECTION ( 'NONE',  ( 0.000000000000000000, 0.000000000000000000, 1.000000000000000000 ) ) ;
#51773=EDGE_CURVE ( 'NONE', #23032, #53791, #46592, .T. ) ;
#51783=CARTESIAN_POINT ( 'NONE',  ( 15.55634918610409656, 36.11269837220803680, 85.00100000000000477 ) ) ;
#51795=DIRECTION ( 'NONE',  ( -0.000000000000000000, -1.000000000000000000, -0.000000000000000000 ) ) ;
#51806=DIRECTION ( 'NONE',  ( 1.000000000000000000, 0.000000000000000000, 0.000000000000000000 ) ) ;
#51826=EDGE_CURVE ( 'NONE', #66496, #4596, #67723, .T. ) ;
#51845=EDGE_CURVE ( 'NONE', #67865, #53174, #34683, .T. ) ;
#51846=ORIENTED_EDGE ( 'NONE', *, *, #49887, .T. ) ;
#51852=ORIENTED_EDGE ( 'NONE', *, *, #15498, .T. ) ;
#51889=DIRECTION ( 'NONE',  ( -0.000000000000000000, -1.000000000000000000, -0.000000000000000000 ) ) ;
#51908=ADVANCED_FACE ( 'NONE', ( #34333 ), #35714, .F. ) ;
#51926=EDGE_CURVE ( 'NONE', #34612, #50750, #42014, .T. ) ;
#51932=VERTEX_POINT ( 'NONE', #47966 ) ;
#51955=EDGE_CURVE ( 'NONE', #5719, #52465, #36397, .T. ) ;
#51969=DIRECTION ( 'NONE',  ( 1.000000000000000000, 0.000000000000000000, 0.000000000000000000 ) ) ;
#51981=ORIENTED_EDGE ( 'NONE', *, *, #5307, .F. ) ;
#51988=VECTOR ( 'NONE', #66929, 1000.000000000000000 ) ;
#51990=EDGE_LOOP ( 'NONE', ( #14251, #61370, #67660, #60470 ) ) ;
#52091=AXIS2_PLACEMENT_3D ( 'NONE', #38764, #59845, #55626 ) ;
#52093=EDGE_CURVE ( 'NONE', #41218, #22868, #41251, .T. ) ;
#52125=DIRECTION ( 'NONE',  ( -0.000000000000000000, -0.000000000000000000, -1.000000000000000000 ) ) ;
#52146=ORIENTED_EDGE ( 'NONE', *, *, #55443, .F. ) ;
#52150=DIRECTION ( 'NONE',  ( 0.000000000000000000, 1.000000000000000000, 0.000000000000000000 ) ) ;
#52171=DIRECTION ( 'NONE',  ( 0.000000000000000000, 0.000000000000000000, 1.000000000000000000 ) ) ;
#52174=DIRECTION ( 'NONE',  ( -0.000000000000000000, -0.000000000000000000, -1.000000000000000000 ) ) ;
#52191=VECTOR ( 'NONE', #62199, 1000.000000000000000 ) ;
#52202=CARTESIAN_POINT ( 'NONE',  ( 31.11269837220806522, 4.999999999999936939, 0.000000000000000000 ) ) ;
#52217=EDGE_LOOP ( 'NONE', ( #68830, #56707, #33982, #65800 ) ) ;
#52236=AXIS2_PLACEMENT_3D ( 'NONE', #38582, #37537, #33326 ) ;
#52243=ADVANCED_FACE ( 'NONE', ( #40128 ), #66189, .F. ) ;
#52260=CARTESIAN_POINT ( 'NONE',  ( 10.55634918610406281, 15.55634918610400241, 2.000000000000000000 ) ) ;
#52272=ORIENTED_EDGE ( 'NONE', *, *, #11992, .T. ) ;
#52273=VERTEX_POINT ( 'NONE', #55963 ) ;
#52286=DIRECTION ( 'NONE',  ( -0.000000000000000000, -0.000000000000000000, -1.000000000000000000 ) ) ;
#52299=EDGE_LOOP ( 'NONE', ( #68752, #4037, #37737, #48898 ) ) ;
#52302=ORIENTED_EDGE ( 'NONE', *, *, #58330, .T. ) ;
#52309=ORIENTED_EDGE ( 'NONE', *, *, #27368, .T. ) ;
#52310=ORIENTED_EDGE ( 'NONE', *, *, #3981, .T. ) ;
#52378=DIRECTION ( 'NONE',  ( -0.000000000000000000, -1.000000000000000000, -0.000000000000000000 ) ) ;
#52390=EDGE_CURVE ( 'NONE', #8516, #45779, #38647, .T. ) ;
#52411=EDGE_CURVE ( 'NONE', #32718, #4563, #31986, .T. ) ;
#52412=EDGE_LOOP ( 'NONE', ( #25334, #60504, #24914, #39337 ) ) ;
#52421=DIRECTION ( 'NONE',  ( -0.000000000000000000, -1.000000000000000000, -0.000000000000000000 ) ) ;
#52435=ADVANCED_FACE ( 'NONE', ( #54098 ), #6635, .F. ) ;
#52465=VERTEX_POINT ( 'NONE', #53417 ) ;
#52475=ORIENTED_EDGE ( 'NONE', *, *, #24778, .T. ) ;
#52485=EDGE_CURVE ( 'NONE', #36200, #60290, #666, .T. ) ;
#52505=CARTESIAN_POINT ( 'NONE',  ( -15.55634918610408945, -26.11269837220804035, 0.000000000000000000 ) ) ;
#52522=CARTESIAN_POINT ( 'NONE',  ( 31.11269837220800127, -31.11269837220812562, 85.00100000000000477 ) ) ;
#52548=EDGE_CURVE ( 'NONE', #35180, #1235, #24218, .T. ) ;
#52550=CARTESIAN_POINT ( 'NONE',  ( 26.11269837220803325, -10.55634918610409656, 2.000000000000001776 ) ) ;
#52574=VECTOR ( 'NONE', #22331, 1000.000000000000000 ) ;
#52576=CARTESIAN_POINT ( 'NONE',  ( -20.55634918610408945, -26.11269837220804035, 2.000000000000001776 ) ) ;
#52583=ORIENTED_EDGE ( 'NONE', *, *, #53979, .T. ) ;
#52585=EDGE_LOOP ( 'NONE', ( #52475, #55422, #22007, #9519 ) ) ;
#52591=FACE_OUTER_BOUND ( 'NONE', #1021, .T. ) ;
#52605=DIRECTION ( 'NONE',  ( -0.000000000000000000, -0.000000000000000000, -1.000000000000000000 ) ) ;
#52620=LINE ( 'NONE', #14992, #38690 ) ;
#52726=ORIENTED_EDGE ( 'NONE', *, *, #22875, .T. ) ;
#52739=ORIENTED_EDGE ( 'NONE', *, *, #3817, .F. ) ;
#52775=AXIS2_PLACEMENT_3D ( 'NONE', #66955, #18752, #51110 ) ;
#52800=ADVANCED_FACE ( 'NONE', ( #7617 ), #2333, .F. ) ;
#52804=EDGE_CURVE ( 'NONE', #12488, #22095, #7950, .T. ) ;
#52807=EDGE_CURVE ( 'NONE', #51157, #33219, #37019, .T. ) ;
#52811=DIRECTION ( 'NONE',  ( 0.000000000000000000, -1.000000000000000000, 0.000000000000000000 ) ) ;
#52835=EDGE_LOOP ( 'NONE', ( #18367, #14030, #8206, #58365 ) ) ;
#52843=CARTESIAN_POINT ( 'NONE',  ( -31.11269837220809364, -10.55634918610397932, 85.00100000000000477 ) ) ;
#52859=CARTESIAN_POINT ( 'NONE',  ( -15.55634918610403439, 2.818925648462311528E-14, 2.000000000000001776 ) ) ;
#52891=ORIENTED_EDGE ( 'NONE', *, *, #11992, .F. ) ;
#52902=LINE ( 'NONE', #4048, #19646 ) ;
#52918=DIRECTION ( 'NONE',  ( 0.000000000000000000, -0.000000000000000000, -1.000000000000000000 ) ) ;
#52919=VECTOR ( 'NONE', #23298, 1000.000000000000000 ) ;
#52928=DIRECTION ( 'NONE',  ( 1.000000000000000000, -0.000000000000000000, -0.000000000000000000 ) ) ;
#52930=CARTESIAN_POINT ( 'NONE',  ( 15.55634918610396511, -41.66904755831214402, 0.000000000000000000 ) ) ;
#52939=VECTOR ( 'NONE', #39436, 1000.000000000000000 ) ;
#52950=ORIENTED_EDGE ( 'NONE', *, *, #28862, .F. ) ;
#52957=DIRECTION ( 'NONE',  ( -0.000000000000000000, -0.000000000000000000, -1.000000000000000000 ) ) ;
#52966=DIRECTION ( 'NONE',  ( -1.000000000000000000, 0.000000000000000000, 0.000000000000000000 ) ) ;
#52976=EDGE_CURVE ( 'NONE', #47695, #38528, #21393, .T. ) ;
#52986=DIRECTION ( 'NONE',  ( -0.000000000000000000, -0.000000000000000000, -1.000000000000000000 ) ) ;
#52990=LINE ( 'NONE', #38556, #17580 ) ;
#53010=ORIENTED_EDGE ( 'NONE', *, *, #36051, .F. ) ;
#53029=ORIENTED_EDGE ( 'NONE', *, *, #32611, .F. ) ;
#53048=LINE ( 'NONE', #58002, #5280 ) ;
#53075=PLANE ( 'NONE',  #53422 ) ;
#53080=DIRECTION ( 'NONE',  ( -1.000000000000000000, 0.000000000000000000, 0.000000000000000000 ) ) ;
#53084=PLANE ( 'NONE',  #4192 ) ;
#53094=EDGE_CURVE ( 'NONE', #8293, #46372, #67164, .T. ) ;
#53096=DIRECTION ( 'NONE',  ( 0.000000000000000000, -1.000000000000000000, 0.000000000000000000 ) ) ;
#53104=ORIENTED_EDGE ( 'NONE', *, *, #46533, .T. ) ;
#53111=EDGE_CURVE ( 'NONE', #59242, #38638, #66813, .T. ) ;
#53125=CIRCLE ( 'NONE', #3742, 66.50000000000000000 ) ;
#53142=CARTESIAN_POINT ( 'NONE',  ( 46.66904755831210139, -9.150666335777657423E-14, 2.000000000000001776 ) ) ;
#53146=EDGE_CURVE ( 'NONE', #56869, #67388, #14017, .T. ) ;
#53174=VERTEX_POINT ( 'NONE', #67841 ) ;
#53175=VECTOR ( 'NONE', #57464, 1000.000000000000000 ) ;
#53178=DIRECTION ( 'NONE',  ( 0.000000000000000000, 0.000000000000000000, -1.000000000000000000 ) ) ;
#53186=DIRECTION ( 'NONE',  ( 1.000000000000000000, 0.000000000000000000, 0.000000000000000000 ) ) ;
#53187=CARTESIAN_POINT ( 'NONE',  ( 46.66904755831212981, 15.55634918610394379, 0.000000000000000000 ) ) ;
#53196=LINE ( 'NONE', #63085, #37466 ) ;
#53213=DIRECTION ( 'NONE',  ( -0.000000000000000000, -0.000000000000000000, -1.000000000000000000 ) ) ;
#53218=AXIS2_PLACEMENT_3D ( 'NONE', #67934, #3219, #67581 ) ;
#53229=CARTESIAN_POINT ( 'NONE',  ( -74.99999999999998579, 9.184850993605147156E-15, 25.00000000000007816 ) ) ;
#53232=VECTOR ( 'NONE', #55278, 1000.000000000000000 ) ;
#53233=ORIENTED_EDGE ( 'NONE', *, *, #53338, .T. ) ;
#53294=ORIENTED_EDGE ( 'NONE', *, *, #44284, .T. ) ;
#53295=CARTESIAN_POINT ( 'NONE',  ( 26.11269837220812562, 36.11269837220800838, 85.00100000000000477 ) ) ;
#53303=EDGE_LOOP ( 'NONE', ( #52302, #61588, #28269, #28578 ) ) ;
#53305=FACE_BOUND ( 'NONE', #60069, .T. ) ;
#53338=EDGE_CURVE ( 'NONE', #62136, #36801, #48763, .T. ) ;
#53363=ORIENTED_EDGE ( 'NONE', *, *, #54690, .F. ) ;
#53364=VECTOR ( 'NONE', #67901, 1000.000000000000000 ) ;
#53417=CARTESIAN_POINT ( 'NONE',  ( -31.11269837220812207, -26.11269837220801193, 0.000000000000000000 ) ) ;
#53420=EDGE_LOOP ( 'NONE', ( #62543, #61172, #45389, #38614 ) ) ;
#53422=AXIS2_PLACEMENT_3D ( 'NONE', #69270, #27039, #16145 ) ;
#53468=EDGE_LOOP ( 'NONE', ( #47400, #9183, #9284, #62089 ) ) ;
#53506=CARTESIAN_POINT ( 'NONE',  ( 26.11269837220806167, 4.999999999999936939, 85.00100000000000477 ) ) ;
#53535=CARTESIAN_POINT ( 'NONE',  ( -46.66904755831212981, -15.55634918610397222, 0.000000000000000000 ) ) ;
#53552=ORIENTED_EDGE ( 'NONE', *, *, #20114, .T. ) ;
#53562=VECTOR ( 'NONE', #66817, 1000.000000000000000 ) ;
#53566=AXIS2_PLACEMENT_3D ( 'NONE', #60679, #45538, #34307 ) ;
#53581=VERTEX_POINT ( 'NONE', #63503 ) ;
#53622=CARTESIAN_POINT ( 'NONE',  ( 0.000000000000000000, 0.000000000000000000, 0.000000000000000000 ) ) ;
#53629=LINE ( 'NONE', #23034, #55193 ) ;
#53654=EDGE_LOOP ( 'NONE', ( #9384, #6312, #24284, #50810 ) ) ;
#53661=VECTOR ( 'NONE', #882, 1000.000000000000000 ) ;
#53685=ADVANCED_FACE ( 'NONE', ( #10630 ), #9618, .F. ) ;
#53691=ORIENTED_EDGE ( 'NONE', *, *, #16349, .F. ) ;
#53707=LINE ( 'NONE', #64274, #23017 ) ;
#53709=CARTESIAN_POINT ( 'NONE',  ( 10.55634918610409656, 31.11269837220803325, 85.00100000000000477 ) ) ;
#53714=VERTEX_POINT ( 'NONE', #58145 ) ;
#53753=AXIS2_PLACEMENT_3D ( 'NONE', #61369, #3322, #8949 ) ;
#53757=EDGE_CURVE ( 'NONE', #33258, #913, #30727, .T. ) ;
#53759=CARTESIAN_POINT ( 'NONE',  ( 2.905661822261151883E-14, 15.55634918610403084, 85.00100000000000477 ) ) ;
#53791=VERTEX_POINT ( 'NONE', #42311 ) ;
#53805=CARTESIAN_POINT ( 'NONE',  ( 26.11269837220803325, -15.55634918610409656, 2.000000000000000000 ) ) ;
#53812=EDGE_CURVE ( 'NONE', #15169, #40853, #60217, .T. ) ;
#53816=VERTEX_POINT ( 'NONE', #12035 ) ;
#53824=ORIENTED_EDGE ( 'NONE', *, *, #53111, .F. ) ;
#53829=CARTESIAN_POINT ( 'NONE',  ( -15.55634918610400597, 15.55634918610405748, 0.000000000000000000 ) ) ;
#53834=VERTEX_POINT ( 'NONE', #81 ) ;
#53853=ORIENTED_EDGE ( 'NONE', *, *, #3014, .F. ) ;
#53881=DIRECTION ( 'NONE',  ( 0.000000000000000000, 0.000000000000000000, -1.000000000000000000 ) ) ;
#53885=DIRECTION ( 'NONE',  ( 0.000000000000000000, 1.000000000000000000, -0.000000000000000000 ) ) ;
#53888=DIRECTION ( 'NONE',  ( 1.000000000000000000, -0.000000000000000000, -0.000000000000000000 ) ) ;
#53909=DIRECTION ( 'NONE',  ( -1.000000000000000000, 0.000000000000000000, 0.000000000000000000 ) ) ;
#53914=CARTESIAN_POINT ( 'NONE',  ( 10.55634918610396511, -46.66904755831214402, 2.000000000000001776 ) ) ;
#53918=VERTEX_POINT ( 'NONE', #430 ) ;
#53924=CARTESIAN_POINT ( 'NONE',  ( 31.11269837220803325, -15.55634918610409656, 85.00100000000000477 ) ) ;
#53955=CARTESIAN_POINT ( 'NONE',  ( 26.11269837220809364, 20.55634918610396866, 85.00100000000000477 ) ) ;
#53961=LINE ( 'NONE', #13523, #39485 ) ;
#53979=EDGE_CURVE ( 'NONE', #22403, #192, #53125, .T. ) ;
#54008=ORIENTED_EDGE ( 'NONE', *, *, #62963, .F. ) ;
#54013=DIRECTION ( 'NONE',  ( 0.000000000000000000, -1.000000000000000000, 0.000000000000000000 ) ) ;
#54018=CARTESIAN_POINT ( 'NONE',  ( 26.11269837220812562, 31.11269837220800483, 85.00100000000000477 ) ) ;
#54020=CARTESIAN_POINT ( 'NONE',  ( -15.55634918610396866, 36.11269837220808654, 2.000000000000001776 ) ) ;
#54031=DIRECTION ( 'NONE',  ( -0.000000000000000000, -0.000000000000000000, -1.000000000000000000 ) ) ;
#54035=ORIENTED_EDGE ( 'NONE', *, *, #67362, .F. ) ;
#54043=DIRECTION ( 'NONE',  ( -0.000000000000000000, -0.000000000000000000, -1.000000000000000000 ) ) ;
#54065=DIRECTION ( 'NONE',  ( -1.000000000000000000, 0.000000000000000000, 0.000000000000000000 ) ) ;
#54070=VECTOR ( 'NONE', #23664, 1000.000000000000000 ) ;
#54073=ORIENTED_EDGE ( 'NONE', *, *, #51826, .F. ) ;
#54076=EDGE_LOOP ( 'NONE', ( #46402, #65065, #5981, #59264 ) ) ;
#54098=FACE_OUTER_BOUND ( 'NONE', #38982, .T. ) ;
#54110=VECTOR ( 'NONE', #4105, 1000.000000000000000 ) ;
#54115=AXIS2_PLACEMENT_3D ( 'NONE', #44322, #65447, #49590 ) ;
#54127=EDGE_CURVE ( 'NONE', #54421, #48274, #37548, .T. ) ;
#54133=ORIENTED_EDGE ( 'NONE', *, *, #25292, .F. ) ;
#54143=VERTEX_POINT ( 'NONE', #57979 ) ;
#54150=EDGE_CURVE ( 'NONE', #66496, #9968, #26317, .T. ) ;
#54164=AXIS2_PLACEMENT_3D ( 'NONE', #14347, #30517, #61820 ) ;
#54173=CARTESIAN_POINT ( 'NONE',  ( 10.55634918610406281, 15.55634918610400241, 85.00100000000000477 ) ) ;
#54196=DIRECTION ( 'NONE',  ( 0.000000000000000000, 0.000000000000000000, -1.000000000000000000 ) ) ;
#54197=LINE ( 'NONE', #64778, #17474 ) ;
#54200=DIRECTION ( 'NONE',  ( -1.000000000000000000, 0.000000000000000000, 0.000000000000000000 ) ) ;
#54230=CARTESIAN_POINT ( 'NONE',  ( -15.55634918610411077, -41.66904755831209428, 85.00100000000000477 ) ) ;
#54247=FACE_OUTER_BOUND ( 'NONE', #36898, .T. ) ;
#54251=CARTESIAN_POINT ( 'NONE',  ( 0.000000000000000000, 0.000000000000000000, 2.000000000000001776 ) ) ;
#54255=CARTESIAN_POINT ( 'NONE',  ( 31.11269837220809364, 15.55634918610396866, 0.000000000000000000 ) ) ;
#54272=EDGE_CURVE ( 'NONE', #7128, #59178, #55463, .T. ) ;
#54278=EDGE_CURVE ( 'NONE', #57346, #26420, #33682, .T. ) ;
#54284=PRESENTATION_STYLE_ASSIGNMENT (( #33567 ) ) ;
#54291=ORIENTED_EDGE ( 'NONE', *, *, #36279, .T. ) ;
#54324=VECTOR ( 'NONE', #41602, 1000.000000000000000 ) ;
#54326=VECTOR ( 'NONE', #33850, 1000.000000000000000 ) ;
#54344=CARTESIAN_POINT ( 'NONE',  ( 46.66904755831212981, 15.55634918610394379, 2.000000000000001776 ) ) ;
#54356=EDGE_CURVE ( 'NONE', #56697, #48044, #49830, .T. ) ;
#54370=CARTESIAN_POINT ( 'NONE',  ( -5.000000000000026645, -10.55634918610403439, 2.000000000000001776 ) ) ;
#54371=VECTOR ( 'NONE', #4927, 1000.000000000000000 ) ;
#54395=DIRECTION ( 'NONE',  ( -0.000000000000000000, -0.000000000000000000, -1.000000000000000000 ) ) ;
#54415=CARTESIAN_POINT ( 'NONE',  ( 0.000000000000000000, 0.000000000000000000, 2.000000000000001776 ) ) ;
#54421=VERTEX_POINT ( 'NONE', #9025 ) ;
#54435=DIRECTION ( 'NONE',  ( 1.000000000000000000, 0.000000000000000000, 0.000000000000000000 ) ) ;
#54443=ORIENTED_EDGE ( 'NONE', *, *, #39883, .F. ) ;
#54474=CARTESIAN_POINT ( 'NONE',  ( 41.66904755831212981, 15.55634918610394379, 2.000000000000000000 ) ) ;
#54489=DIRECTION ( 'NONE',  ( -0.000000000000000000, -0.000000000000000000, -1.000000000000000000 ) ) ;
#54490=VERTEX_POINT ( 'NONE', #4765 ) ;
#54526=CARTESIAN_POINT ( 'NONE',  ( 73.43826238111391547, 0.000000000000000000, 26.24939009510892518 ) ) ;
#54532=LINE ( 'NONE', #42604, #41753 ) ;
#54536=DIRECTION ( 'NONE',  ( 0.000000000000000000, 1.000000000000000000, -0.000000000000000000 ) ) ;
#54543=FACE_OUTER_BOUND ( 'NONE', #63287, .T. ) ;
#54565=EDGE_CURVE ( 'NONE', #59604, #44250, #44834, .T. ) ;
#54601=ORIENTED_EDGE ( 'NONE', *, *, #42234, .T. ) ;
#54602=EDGE_CURVE ( 'NONE', #5602, #23803, #6032, .T. ) ;
#54608=CARTESIAN_POINT ( 'NONE',  ( 15.55634918610406103, 20.55634918610400064, 0.000000000000000000 ) ) ;
#54680=ORIENTED_EDGE ( 'NONE', *, *, #39883, .T. ) ;
#54683=VECTOR ( 'NONE', #33579, 1000.000000000000000 ) ;
#54686=EDGE_CURVE ( 'NONE', #53714, #45779, #56422, .T. ) ;
#54690=EDGE_CURVE ( 'NONE', #66166, #33134, #18793, .T. ) ;
#54699=EDGE_CURVE ( 'NONE', #53834, #3914, #29693, .T. ) ;
#54708=VERTEX_POINT ( 'NONE', #9274 ) ;
#54722=EDGE_LOOP ( 'NONE', ( #16136, #10276, #24912, #8688 ) ) ;
#54740=CARTESIAN_POINT ( 'NONE',  ( -15.55634918610408945, -31.11269837220804035, 2.000000000000001776 ) ) ;
#54789=EDGE_CURVE ( 'NONE', #14795, #30095, #68698, .T. ) ;
#54810=CARTESIAN_POINT ( 'NONE',  ( 0.000000000000000000, 0.000000000000000000, 85.00000000000000000 ) ) ;
#54817=LINE ( 'NONE', #38652, #64437 ) ;
#54821=LINE ( 'NONE', #6643, #18641 ) ;
#54834=FACE_OUTER_BOUND ( 'NONE', #7425, .T. ) ;
#54850=EDGE_CURVE ( 'NONE', #16148, #23177, #20510, .T. ) ;
#54860=EDGE_CURVE ( 'NONE', #35681, #60290, #53196, .T. ) ;
#54863=DIRECTION ( 'NONE',  ( 0.000000000000000000, 0.000000000000000000, 1.000000000000000000 ) ) ;
#54865=AXIS2_PLACEMENT_3D ( 'NONE', #54230, #16952, #38420 ) ;
#54872=LINE ( 'NONE', #7405, #11694 ) ;
#54878=DIRECTION ( 'NONE',  ( 0.000000000000000000, 0.000000000000000000, 1.000000000000000000 ) ) ;
#54888=ORIENTED_EDGE ( 'NONE', *, *, #17807, .T. ) ;
#54914=ORIENTED_EDGE ( 'NONE', *, *, #12242, .T. ) ;
#54915=ORIENTED_EDGE ( 'NONE', *, *, #19934, .T. ) ;
#54931=DIRECTION ( 'NONE',  ( -1.000000000000000000, 0.000000000000000000, 0.000000000000000000 ) ) ;
#54955=EDGE_CURVE ( 'NONE', #22638, #22983, #1141, .T. ) ;
#54956=ORIENTED_EDGE ( 'NONE', *, *, #46561, .F. ) ;
#54960=EDGE_CURVE ( 'NONE', #58410, #16538, #22592, .T. ) ;
#54963=ADVANCED_FACE ( 'NONE', ( #34897 ), #56005, .F. ) ;
#54986=EDGE_LOOP ( 'NONE', ( #16341, #33012, #7874, #4471 ) ) ;
#54996=DIRECTION ( 'NONE',  ( 0.000000000000000000, 1.000000000000000000, -0.000000000000000000 ) ) ;
#55020=EDGE_CURVE ( 'NONE', #14714, #62926, #24690, .T. ) ;
#55035=ORIENTED_EDGE ( 'NONE', *, *, #18118, .F. ) ;
#55039=EDGE_LOOP ( 'NONE', ( #50309, #4201, #3356, #32133 ) ) ;
#55046=EDGE_CURVE ( 'NONE', #11058, #37117, #55641, .T. ) ;
#55081=DIRECTION ( 'NONE',  ( 1.000000000000000000, 0.000000000000000000, 0.000000000000000000 ) ) ;
#55118=CARTESIAN_POINT ( 'NONE',  ( -20.55634918610396866, 31.11269837220809009, 0.000000000000000000 ) ) ;
#55124=CARTESIAN_POINT ( 'NONE',  ( 10.55634918610403084, 4.999999999999969802, 2.000000000000001776 ) ) ;
#55128=VERTEX_POINT ( 'NONE', #53805 ) ;
#55136=ORIENTED_EDGE ( 'NONE', *, *, #49210, .T. ) ;
#55140=FACE_OUTER_BOUND ( 'NONE', #36183, .T. ) ;
#55146=DIRECTION ( 'NONE',  ( 1.000000000000000000, 0.000000000000000000, 0.000000000000000000 ) ) ;
#55149=EDGE_LOOP ( 'NONE', ( #52583, #21388, #67791, #38564 ) ) ;
#55154=DIRECTION ( 'NONE',  ( 0.000000000000000000, 0.000000000000000000, 1.000000000000000000 ) ) ;
#55179=VERTEX_POINT ( 'NONE', #17588 ) ;
#55193=VECTOR ( 'NONE', #5791, 1000.000000000000000 ) ;
#55218=ORIENTED_EDGE ( 'NONE', *, *, #67027, .F. ) ;
#55227=CARTESIAN_POINT ( 'NONE',  ( 15.55634918610400241, -15.55634918610406103, 0.000000000000000000 ) ) ;
#55235=CARTESIAN_POINT ( 'NONE',  ( -31.11269837220809364, -15.55634918610397754, 85.00100000000000477 ) ) ;
#55248=DIRECTION ( 'NONE',  ( 0.000000000000000000, 0.000000000000000000, 1.000000000000000000 ) ) ;
#55249=ADVANCED_FACE ( 'NONE', ( #28130 ), #43252, .F. ) ;
#55257=ADVANCED_FACE ( 'NONE', ( #39053 ), #66778, .F. ) ;
#55259=DIRECTION ( 'NONE',  ( 1.000000000000000000, 0.000000000000000000, 0.000000000000000000 ) ) ;
#55260=VECTOR ( 'NONE', #47433, 1000.000000000000000 ) ;
#55278=DIRECTION ( 'NONE',  ( -0.000000000000000000, -1.000000000000000000, -0.000000000000000000 ) ) ;
#55282=CARTESIAN_POINT ( 'NONE',  ( 15.55634918610400241, -15.55634918610406103, 2.000000000000001776 ) ) ;
#55295=AXIS2_PLACEMENT_3D ( 'NONE', #46323, #57239, #15012 ) ;
#55314=LINE ( 'NONE', #5729, #63493 ) ;
#55325=ORIENTED_EDGE ( 'NONE', *, *, #21210, .T. ) ;
#55379=EDGE_LOOP ( 'NONE', ( #45145, #26287, #20440, #21478 ) ) ;
#55386=DIRECTION ( 'NONE',  ( 0.000000000000000000, 0.000000000000000000, 1.000000000000000000 ) ) ;
#55392=LINE ( 'NONE', #7221, #45949 ) ;
#55402=VECTOR ( 'NONE', #26743, 1000.000000000000000 ) ;
#55422=ORIENTED_EDGE ( 'NONE', *, *, #55423, .T. ) ;
#55423=EDGE_CURVE ( 'NONE', #54490, #33627, #29029, .T. ) ;
#55438=LINE ( 'NONE', #7271, #29798 ) ;
#55442=ADVANCED_FACE ( 'NONE', ( #50122 ), #44842, .F. ) ;
#55443=EDGE_CURVE ( 'NONE', #57346, #32720, #49751, .T. ) ;
#55463=LINE ( 'NONE', #66046, #31805 ) ;
#55484=ORIENTED_EDGE ( 'NONE', *, *, #24503, .F. ) ;
#55493=FACE_BOUND ( 'NONE', #20376, .T. ) ;
#55545=CARTESIAN_POINT ( 'NONE',  ( 15.55634918610403261, 4.999999999999969802, 85.00100000000000477 ) ) ;
#55592=EDGE_CURVE ( 'NONE', #12059, #32583, #51168, .T. ) ;
#55603=CARTESIAN_POINT ( 'NONE',  ( 31.11269837220812562, 31.11269837220800483, 2.000000000000001776 ) ) ;
#55610=AXIS2_PLACEMENT_3D ( 'NONE', #58181, #827, #63810 ) ;
#55617=LINE ( 'NONE', #60549, #9723 ) ;
#55624=LINE ( 'NONE', #2517, #46904 ) ;
#55626=DIRECTION ( 'NONE',  ( 0.000000000000000000, 0.000000000000000000, 1.000000000000000000 ) ) ;
#55641=LINE ( 'NONE', #7814, #13883 ) ;
#55658=LINE ( 'NONE', #7489, #57960 ) ;
#55668=LINE ( 'NONE', #9130, #69096 ) ;
#55693=AXIS2_PLACEMENT_3D ( 'NONE', #11722, #38463, #5748 ) ;
#55694=LINE ( 'NONE', #33900, #18312 ) ;
#55744=VERTEX_POINT ( 'NONE', #15941 ) ;
#55793=LINE ( 'NONE', #66708, #22830 ) ;
#55794=ORIENTED_EDGE ( 'NONE', *, *, #2401, .T. ) ;
#55798=AXIS2_PLACEMENT_3D ( 'NONE', #46335, #51969, #29825 ) ;
#55848=VECTOR ( 'NONE', #59833, 1000.000000000000000 ) ;
#55854=EDGE_LOOP ( 'NONE', ( #51227, #22213, #17142, #5912 ) ) ;
#55857=EDGE_CURVE ( 'NONE', #16162, #51932, #66241, .T. ) ;
#55879=ORIENTED_EDGE ( 'NONE', *, *, #49858, .T. ) ;
#55883=PLANE ( 'NONE',  #49814 ) ;
#55892=DIRECTION ( 'NONE',  ( 1.000000000000000000, 0.000000000000000000, 0.000000000000000000 ) ) ;
#55910=LINE ( 'NONE', #29512, #35716 ) ;
#55911=DIRECTION ( 'NONE',  ( -1.000000000000000000, 0.000000000000000000, 0.000000000000000000 ) ) ;
#55916=CARTESIAN_POINT ( 'NONE',  ( -5.000000000000026645, -15.55634918610403616, 85.00100000000000477 ) ) ;
#55918=AXIS2_PLACEMENT_3D ( 'NONE', #21168, #6370, #11633 ) ;
#55921=ORIENTED_EDGE ( 'NONE', *, *, #26667, .F. ) ;
#55963=CARTESIAN_POINT ( 'NONE',  ( 31.11269837220800127, -26.11269837220812562, 0.000000000000000000 ) ) ;
#55984=LINE ( 'NONE', #7796, #66002 ) ;
#56005=PLANE ( 'NONE',  #31858 ) ;
#56017=CARTESIAN_POINT ( 'NONE',  ( -46.66904755831210139, 5.000000000000066613, 0.000000000000000000 ) ) ;
#56041=CARTESIAN_POINT ( 'NONE',  ( 10.55634918610411432, 46.66904755831205875, 0.000000000000000000 ) ) ;
#56106=FACE_OUTER_BOUND ( 'NONE', #576, .T. ) ;
#56113=EDGE_LOOP ( 'NONE', ( #2216, #51846, #69043, #19050 ) ) ;
#56118=DIRECTION ( 'NONE',  ( -1.000000000000000000, 0.000000000000000000, 0.000000000000000000 ) ) ;
#56132=DIRECTION ( 'NONE',  ( 0.000000000000000000, -0.000000000000000000, -1.000000000000000000 ) ) ;
#56143=CARTESIAN_POINT ( 'NONE',  ( 15.55634918610396511, -46.66904755831214402, 2.000000000000001776 ) ) ;
#56149=EDGE_LOOP ( 'NONE', ( #65647, #13365, #61084, #14228 ) ) ;
#56151=CARTESIAN_POINT ( 'NONE',  ( 10.55634918610400419, -15.55634918610406103, 85.00100000000000477 ) ) ;
#56157=EDGE_CURVE ( 'NONE', #8745, #7128, #34456, .T. ) ;
#56172=ORIENTED_EDGE ( 'NONE', *, *, #47087, .F. ) ;
#56204=LINE ( 'NONE', #34427, #57572 ) ;
#56222=FACE_OUTER_BOUND ( 'NONE', #18722, .T. ) ;
#56228=LINE ( 'NONE', #12282, #6130 ) ;
#56240=VERTEX_POINT ( 'NONE', #9042 ) ;
#56251=LINE ( 'NONE', #45352, #2498 ) ;
#56257=CARTESIAN_POINT ( 'NONE',  ( 41.66904755831210849, -9.150666335777657423E-14, 2.000000000000001776 ) ) ;
#56265=VERTEX_POINT ( 'NONE', #29801 ) ;
#56295=CARTESIAN_POINT ( 'NONE',  ( 10.55634918610409656, 31.11269837220803325, 85.00100000000000477 ) ) ;
#56296=EDGE_CURVE ( 'NONE', #30795, #38817, #2723, .T. ) ;
#56304=EDGE_CURVE ( 'NONE', #19283, #66816, #29752, .T. ) ;
#56320=VECTOR ( 'NONE', #6398, 1000.000000000000000 ) ;
#56331=CARTESIAN_POINT ( 'NONE',  ( 0.000000000000000000, 0.000000000000000000, 26.24939009510892518 ) ) ;
#56342=EDGE_LOOP ( 'NONE', ( #28507, #32327, #33271, #21059 ) ) ;
#56359=PRODUCT ( 'back cover', 'back cover', '', ( #9023 ) ) ;
#56361=EDGE_CURVE ( 'NONE', #47170, #27210, #20276, .T. ) ;
#56370=ORIENTED_EDGE ( 'NONE', *, *, #10728, .F. ) ;
#56400=CARTESIAN_POINT ( 'NONE',  ( 46.66904755831210139, -9.150666335777657423E-14, 85.00100000000000477 ) ) ;
#56407=VERTEX_POINT ( 'NONE', #57913 ) ;
#56412=DIRECTION ( 'NONE',  ( 0.000000000000000000, -1.000000000000000000, 0.000000000000000000 ) ) ;
#56421=VECTOR ( 'NONE', #6073, 1000.000000000000000 ) ;
#56422=LINE ( 'NONE', #62749, #7156 ) ;
#56432=CARTESIAN_POINT ( 'NONE',  ( -5.767955557622883589E-14, -31.11269837220806878, 85.00100000000000477 ) ) ;
#56459=CARTESIAN_POINT ( 'NONE',  ( -20.55634918610396866, 31.11269837220809009, 85.00100000000000477 ) ) ;
#56475=FACE_OUTER_BOUND ( 'NONE', #34985, .T. ) ;
#56479=ORIENTED_EDGE ( 'NONE', *, *, #66650, .T. ) ;
#56481=CARTESIAN_POINT ( 'NONE',  ( 31.11269837220806522, -6.375108774214766072E-14, 2.000000000000001776 ) ) ;
#56487=LINE ( 'NONE', #51223, #11265 ) ;
#56495=CARTESIAN_POINT ( 'NONE',  ( 15.55634918610396511, -41.66904755831214402, 0.000000000000000000 ) ) ;
#56496=LINE ( 'NONE', #32193, #5126 ) ;
#56513=ORIENTED_EDGE ( 'NONE', *, *, #5876, .F. ) ;
#56530=ORIENTED_EDGE ( 'NONE', *, *, #5092, .T. ) ;
#56572=DIRECTION ( 'NONE',  ( 1.000000000000000000, 0.000000000000000000, 0.000000000000000000 ) ) ;
#56576=VECTOR ( 'NONE', #21612, 1000.000000000000000 ) ;
#56585=CARTESIAN_POINT ( 'NONE',  ( 15.55634918610397399, -26.11269837220809364, 85.00100000000000477 ) ) ;
#56596=EDGE_CURVE ( 'NONE', #32692, #52465, #43101, .T. ) ;
#56607=DIRECTION ( 'NONE',  ( 0.000000000000000000, 1.000000000000000000, -0.000000000000000000 ) ) ;
#56610=ORIENTED_EDGE ( 'NONE', *, *, #43895, .T. ) ;
#56619=VECTOR ( 'NONE', #15579, 1000.000000000000000 ) ;
#56630=LINE ( 'NONE', #35174, #2783 ) ;
#56647=DIRECTION ( 'NONE',  ( -1.000000000000000000, 0.000000000000000000, 0.000000000000000000 ) ) ;
#56661=FACE_OUTER_BOUND ( 'NONE', #24522, .T. ) ;
#56669=FACE_OUTER_BOUND ( 'NONE', #57868, .T. ) ;
#56687=CARTESIAN_POINT ( 'NONE',  ( 6.375108774214766072E-14, 31.11269837220806167, 2.000000000000001776 ) ) ;
#56696=DIRECTION ( 'NONE',  ( 0.000000000000000000, -0.000000000000000000, -1.000000000000000000 ) ) ;
#56697=VERTEX_POINT ( 'NONE', #37396 ) ;
#56707=ORIENTED_EDGE ( 'NONE', *, *, #20722, .T. ) ;
#56712=AXIS2_PLACEMENT_3D ( 'NONE', #15744, #10808, #5530 ) ;
#56772=CARTESIAN_POINT ( 'NONE',  ( -20.55634918610405748, -10.55634918610400597, 2.000000000000001776 ) ) ;
#56775=VECTOR ( 'NONE', #68734, 1000.000000000000000 ) ;
#56798=CARTESIAN_POINT ( 'NONE',  ( -36.11269837220806522, 5.000000000000056843, 85.00100000000000477 ) ) ;
#56806=VECTOR ( 'NONE', #10009, 1000.000000000000000 ) ;
#56837=DIRECTION ( 'NONE',  ( -1.000000000000000000, 0.000000000000000000, 0.000000000000000000 ) ) ;
#56840=ORIENTED_EDGE ( 'NONE', *, *, #13575, .T. ) ;
#56843=FACE_OUTER_BOUND ( 'NONE', #18230, .T. ) ;
#56852=VERTEX_POINT ( 'NONE', #43364 ) ;
#56856=CYLINDRICAL_SURFACE ( 'NONE', #35383, 66.50000000000000000 ) ;
#56866=LINE ( 'NONE', #47322, #57862 ) ;
#56869=VERTEX_POINT ( 'NONE', #32824 ) ;
#56885=EDGE_CURVE ( 'NONE', #19020, #59151, #55314, .T. ) ;
#56888=CARTESIAN_POINT ( 'NONE',  ( 10.55634918610397577, -31.11269837220809364, 85.00100000000000477 ) ) ;
#56903=DIRECTION ( 'NONE',  ( -0.000000000000000000, -0.000000000000000000, -1.000000000000000000 ) ) ;
#56928=CARTESIAN_POINT ( 'NONE',  ( 31.11269837220809364, 15.55634918610396866, 0.000000000000000000 ) ) ;
#56951=CARTESIAN_POINT ( 'NONE',  ( -20.55634918610403261, 2.818925648462311528E-14, 0.000000000000000000 ) ) ;
#56962=ORIENTED_EDGE ( 'NONE', *, *, #5307, .T. ) ;
#56973=AXIS2_PLACEMENT_3D ( 'NONE', #43802, #17428, #22715 ) ;
#56988=LINE ( 'NONE', #25679, #41710 ) ;
#56996=EDGE_CURVE ( 'NONE', #14102, #35061, #55668, .T. ) ;
#57008=DIRECTION ( 'NONE',  ( 1.000000000000000000, -0.000000000000000000, 0.000000000000000000 ) ) ;
#57011=FACE_OUTER_BOUND ( 'NONE', #42542, .T. ) ;
#57015=LINE ( 'NONE', #61923, #24343 ) ;
#57051=FACE_OUTER_BOUND ( 'NONE', #46630, .T. ) ;
#57068=DIRECTION ( 'NONE',  ( 1.000000000000000000, 0.000000000000000000, -0.000000000000000000 ) ) ;
#57072=EDGE_LOOP ( 'NONE', ( #38746, #21811, #5041, #14119 ) ) ;
#57095=CARTESIAN_POINT ( 'NONE',  ( -15.55634918610403439, 5.000000000000028422, 0.000000000000000000 ) ) ;
#57104=FACE_OUTER_BOUND ( 'NONE', #45919, .T. ) ;
#57137=VERTEX_POINT ( 'NONE', #59710 ) ;
#57139=CARTESIAN_POINT ( 'NONE',  ( 10.55634918610403084, -3.079134169858832593E-14, 0.000000000000000000 ) ) ;
#57143=DIRECTION ( 'NONE',  ( 0.000000000000000000, -1.000000000000000000, 0.000000000000000000 ) ) ;
#57144=CARTESIAN_POINT ( 'NONE',  ( 26.11269837220803325, -15.55634918610409656, 85.00100000000000477 ) ) ;
#57191=DIRECTION ( 'NONE',  ( 0.000000000000000000, -1.000000000000000000, 0.000000000000000000 ) ) ;
#57239=DIRECTION ( 'NONE',  ( 0.000000000000000000, 1.000000000000000000, -0.000000000000000000 ) ) ;
#57246=LINE ( 'NONE', #68489, #21664 ) ;
#57251=PLANE ( 'NONE',  #19963 ) ;
#57320=LINE ( 'NONE', #36211, #41807 ) ;
#57336=EDGE_CURVE ( 'NONE', #69014, #40747, #20622, .T. ) ;
#57338=DIRECTION ( 'NONE',  ( -1.000000000000000000, 0.000000000000000000, 0.000000000000000000 ) ) ;
#57346=VERTEX_POINT ( 'NONE', #63548 ) ;
#57353=CARTESIAN_POINT ( 'NONE',  ( -4.999999999999971578, 15.55634918610403084, 85.00100000000000477 ) ) ;
#57412=DIRECTION ( 'NONE',  ( 0.000000000000000000, 0.000000000000000000, 1.000000000000000000 ) ) ;
#57414=VECTOR ( 'NONE', #96, 1000.000000000000000 ) ;
#57429=ORIENTED_EDGE ( 'NONE', *, *, #50363, .F. ) ;
#57440=PLANE ( 'NONE',  #45007 ) ;
#57464=DIRECTION ( 'NONE',  ( 1.000000000000000000, -0.000000000000000000, -0.000000000000000000 ) ) ;
#57473=CARTESIAN_POINT ( 'NONE',  ( 41.66904755831212981, 20.55634918610394735, 2.000000000000001776 ) ) ;
#57480=CARTESIAN_POINT ( 'NONE',  ( -36.11269837220812207, -26.11269837220801193, 0.000000000000000000 ) ) ;
#57484=LINE ( 'NONE', #43617, #46566 ) ;
#57508=LINE ( 'NONE', #24811, #56775 ) ;
#57515=PLANE ( 'NONE',  #64578 ) ;
#57520=ADVANCED_FACE ( 'NONE', ( #62431 ), #29379, .F. ) ;
#57526=ORIENTED_EDGE ( 'NONE', *, *, #12497, .F. ) ;
#57538=PLANE ( 'NONE',  #8281 ) ;
#57555=CARTESIAN_POINT ( 'NONE',  ( 26.11269837220803325, -15.55634918610409656, 0.000000000000000000 ) ) ;
#57559=CARTESIAN_POINT ( 'NONE',  ( -31.11269837220806878, 5.594483210025202879E-14, 85.00100000000000477 ) ) ;
#57560=CARTESIAN_POINT ( 'NONE',  ( 31.11269837220812562, 36.11269837220800838, 0.000000000000000000 ) ) ;
#57562=ADVANCED_FACE ( 'NONE', ( #34675 ), #67373, .F. ) ;
#57572=VECTOR ( 'NONE', #7335, 1000.000000000000000 ) ;
#57581=VERTEX_POINT ( 'NONE', #19868 ) ;
#57588=FACE_BOUND ( 'NONE', #27245, .T. ) ;
#57595=DIRECTION ( 'NONE',  ( 1.000000000000000000, -0.000000000000000000, 0.000000000000000000 ) ) ;
#57622=LINE ( 'NONE', #41786, #37135 ) ;
#57627=CARTESIAN_POINT ( 'NONE',  ( -7.329206686002009974E-14, -41.66904755831212270, 0.000000000000000000 ) ) ;
#57643=ORIENTED_EDGE ( 'NONE', *, *, #56596, .T. ) ;
#57656=ORIENTED_EDGE ( 'NONE', *, *, #39700, .T. ) ;
#57659=ORIENTED_EDGE ( 'NONE', *, *, #47398, .T. ) ;
#57665=VECTOR ( 'NONE', #57008, 1000.000000000000000 ) ;
#57709=LINE ( 'NONE', #4580, #50175 ) ;
#57724=VECTOR ( 'NONE', #53888, 1000.000000000000000 ) ;
#57742=LINE ( 'NONE', #35940, #558 ) ;
#57745=EDGE_CURVE ( 'NONE', #39519, #10376, #69424, .T. ) ;
#57748=FACE_OUTER_BOUND ( 'NONE', #16819, .T. ) ;
#57784=DIRECTION ( 'NONE',  ( -1.000000000000000000, 0.000000000000000000, 0.000000000000000000 ) ) ;
#57804=EDGE_CURVE ( 'NONE', #59960, #30631, #15961, .T. ) ;
#57813=CARTESIAN_POINT ( 'NONE',  ( -4.999999999999922728, 46.66904755831208718, 2.000000000000001776 ) ) ;
#57835=ORIENTED_EDGE ( 'NONE', *, *, #62086, .T. ) ;
#57862=VECTOR ( 'NONE', #52605, 1000.000000000000000 ) ;
#57868=EDGE_LOOP ( 'NONE', ( #7694, #53233, #25738, #25235 ) ) ;
#57877=DIRECTION ( 'NONE',  ( 0.000000000000000000, 0.000000000000000000, -1.000000000000000000 ) ) ;
#57891=ADVANCED_FACE ( 'NONE', ( #828 ), #33884, .F. ) ;
#57913=CARTESIAN_POINT ( 'NONE',  ( 10.55634918610411432, 51.66904755831205875, 0.000000000000000000 ) ) ;
#57914=ORIENTED_EDGE ( 'NONE', *, *, #61227, .F. ) ;
#57925=ORIENTED_EDGE ( 'NONE', *, *, #41674, .F. ) ;
#57927=PLANE ( 'NONE',  #25041 ) ;
#57934=VERTEX_POINT ( 'NONE', #39168 ) ;
#57960=VECTOR ( 'NONE', #2899, 1000.000000000000000 ) ;
#57975=ADVANCED_FACE ( 'NONE', ( #49687 ), #27902, .F. ) ;
#57976=ORIENTED_EDGE ( 'NONE', *, *, #3399, .F. ) ;
#57979=CARTESIAN_POINT ( 'NONE',  ( 31.11269837220803325, -10.55634918610409656, 0.000000000000000000 ) ) ;
#57995=DIRECTION ( 'NONE',  ( -1.000000000000000000, 0.000000000000000000, 0.000000000000000000 ) ) ;
#58000=VERTEX_POINT ( 'NONE', #62697 ) ;
#58002=CARTESIAN_POINT ( 'NONE',  ( 31.11269837220803325, -10.55634918610409656, 0.000000000000000000 ) ) ;
#58133=VERTEX_POINT ( 'NONE', #20122 ) ;
#58142=FACE_OUTER_BOUND ( 'NONE', #48988, .T. ) ;
#58145=CARTESIAN_POINT ( 'NONE',  ( -4.999999999999922728, 51.66904755831208718, 0.000000000000000000 ) ) ;
#58148=CARTESIAN_POINT ( 'NONE',  ( 7.762887554996211747E-14, 46.66904755831208718, 85.00100000000000477 ) ) ;
#58149=DIRECTION ( 'NONE',  ( 0.000000000000000000, -1.000000000000000000, 0.000000000000000000 ) ) ;
#58162=LINE ( 'NONE', #5385, #57414 ) ;
#58181=CARTESIAN_POINT ( 'NONE',  ( 15.55634918610403261, -3.079134169858832593E-14, 85.00100000000000477 ) ) ;
#58187=PLANE ( 'NONE',  #55693 ) ;
#58214=DIRECTION ( 'NONE',  ( -1.000000000000000000, 0.000000000000000000, 0.000000000000000000 ) ) ;
#58247=DIRECTION ( 'NONE',  ( 1.000000000000000000, -0.000000000000000000, -0.000000000000000000 ) ) ;
#58260=VERTEX_POINT ( 'NONE', #47189 ) ;
#58267=CARTESIAN_POINT ( 'NONE',  ( 0.000000000000000000, 0.000000000000000000, 85.00000000000000000 ) ) ;
#58275=DIRECTION ( 'NONE',  ( 0.000000000000000000, -0.000000000000000000, -1.000000000000000000 ) ) ;
#58298=EDGE_LOOP ( 'NONE', ( #30846, #40237, #67286, #52726 ) ) ;
#58300=ORIENTED_EDGE ( 'NONE', *, *, #62373, .T. ) ;
#58306=CARTESIAN_POINT ( 'NONE',  ( 31.11269837220809364, 15.55634918610396866, 85.00100000000000477 ) ) ;
#58310=DIRECTION ( 'NONE',  ( 0.000000000000000000, 1.000000000000000000, -0.000000000000000000 ) ) ;
#58321=CARTESIAN_POINT ( 'NONE',  ( 15.55634918610396511, -46.66904755831214402, 0.000000000000000000 ) ) ;
#58330=EDGE_CURVE ( 'NONE', #26077, #17896, #65461, .T. ) ;
#58334=AXIS2_PLACEMENT_3D ( 'NONE', #30076, #4710, #40968 ) ;
#58343=ADVANCED_FACE ( 'NONE', ( #17615 ), #33797, .F. ) ;
#58365=ORIENTED_EDGE ( 'NONE', *, *, #29341, .F. ) ;
#58374=EDGE_CURVE ( 'NONE', #23331, #26077, #7060, .T. ) ;
#58385=DIRECTION ( 'NONE',  ( 0.000000000000000000, -0.000000000000000000, -1.000000000000000000 ) ) ;
#58386=CARTESIAN_POINT ( 'NONE',  ( 31.11269837220809364, 15.55634918610396866, 85.00100000000000477 ) ) ;
#58397=ORIENTED_EDGE ( 'NONE', *, *, #60815, .T. ) ;
#58410=VERTEX_POINT ( 'NONE', #1087 ) ;
#58421=EDGE_CURVE ( 'NONE', #21953, #7128, #27458, .T. ) ;
#58432=DIRECTION ( 'NONE',  ( 0.000000000000000000, -1.000000000000000000, 0.000000000000000000 ) ) ;
#58461=ORIENTED_EDGE ( 'NONE', *, *, #49858, .F. ) ;
#58464=CARTESIAN_POINT ( 'NONE',  ( 41.66904755831212981, 15.55634918610394379, 0.000000000000000000 ) ) ;
#58477=ORIENTED_EDGE ( 'NONE', *, *, #14825, .F. ) ;
#58502=ADVANCED_FACE ( 'NONE', ( #22368 ), #65282, .F. ) ;
#58527=ORIENTED_EDGE ( 'NONE', *, *, #17570, .F. ) ;
#58547=VERTEX_POINT ( 'NONE', #25336 ) ;
#58567=ORIENTED_EDGE ( 'NONE', *, *, #58585, .F. ) ;
#58585=EDGE_CURVE ( 'NONE', #39680, #55744, #18145, .T. ) ;
#58589=FACE_BOUND ( 'NONE', #31359, .T. ) ;
#58617=LINE ( 'NONE', #31902, #19686 ) ;
#58638=FACE_OUTER_BOUND ( 'NONE', #10804, .T. ) ;
#58678=ORIENTED_EDGE ( 'NONE', *, *, #15772, .F. ) ;
#58695=AXIS2_PLACEMENT_3D ( 'NONE', #19696, #41162, #30954 ) ;
#58724=CARTESIAN_POINT ( 'NONE',  ( 15.55634918610396511, -41.66904755831214402, 85.00100000000000477 ) ) ;
#58733=DIRECTION ( 'NONE',  ( -1.000000000000000000, 0.000000000000000000, 0.000000000000000000 ) ) ;
#58735=DIRECTION ( 'NONE',  ( 0.000000000000000000, 1.000000000000000000, -0.000000000000000000 ) ) ;
#58746=VECTOR ( 'NONE', #3103, 1000.000000000000000 ) ;
#58748=VECTOR ( 'NONE', #33185, 1000.000000000000000 ) ;
#58771=CARTESIAN_POINT ( 'NONE',  ( 0.000000000000000000, 0.000000000000000000, 26.24939009510892518 ) ) ;
#58776=FACE_OUTER_BOUND ( 'NONE', #53420, .T. ) ;
#58784=LINE ( 'NONE', #53506, #16440 ) ;
#58801=EDGE_CURVE ( 'NONE', #59960, #3346, #8981, .T. ) ;
#58819=DIRECTION ( 'NONE',  ( 0.000000000000000000, 0.000000000000000000, -1.000000000000000000 ) ) ;
#58837=CARTESIAN_POINT ( 'NONE',  ( 15.55634918610403261, 4.999999999999969802, 2.000000000000001776 ) ) ;
#58852=CIRCLE ( 'NONE', #36377, 72.99999999999998579 ) ;
#58854=EDGE_LOOP ( 'NONE', ( #8482, #47639, #64470, #24874 ) ) ;
#58861=CARTESIAN_POINT ( 'NONE',  ( 41.66904755831208007, -10.55634918610412853, 85.00100000000000477 ) ) ;
#58863=ORIENTED_EDGE ( 'NONE', *, *, #23985, .F. ) ;
#58905=DIRECTION ( 'NONE',  ( -0.000000000000000000, -0.000000000000000000, -1.000000000000000000 ) ) ;
#58918=EDGE_LOOP ( 'NONE', ( #28114, #41159, #50704, #32211 ) ) ;
#58934=VERTEX_POINT ( 'NONE', #49000 ) ;
#58938=CARTESIAN_POINT ( 'NONE',  ( 0.000000000000000000, 0.000000000000000000, 2.000000000000000000 ) ) ;
#58979=DIRECTION ( 'NONE',  ( 1.000000000000000000, -0.000000000000000000, 0.000000000000000000 ) ) ;
#58988=PLANE ( 'NONE',  #56712 ) ;
#58994=ADVANCED_FACE ( 'NONE', ( #25428 ), #8552, .F. ) ;
#58995=ADVANCED_FACE ( 'NONE', ( #2579 ), #40547, .F. ) ;
#58998=DIRECTION ( 'NONE',  ( 0.000000000000000000, 1.000000000000000000, -0.000000000000000000 ) ) ;
#59002=ORIENTED_EDGE ( 'NONE', *, *, #53146, .F. ) ;
#59016=CARTESIAN_POINT ( 'NONE',  ( 15.55634918610403261, 4.999999999999969802, 0.000000000000000000 ) ) ;
#59039=ADVANCED_FACE ( 'NONE', ( #19436 ), #13814, .F. ) ;
#59044=LINE ( 'NONE', #9844, #22090 ) ;
#59052=CARTESIAN_POINT ( 'NONE',  ( -46.66904755831210139, 5.000000000000066613, 2.000000000000001776 ) ) ;
#59060=CARTESIAN_POINT ( 'NONE',  ( 15.55634918610403261, -3.079134169858832593E-14, 85.00100000000000477 ) ) ;
#59063=DIRECTION ( 'NONE',  ( 1.000000000000000000, 0.000000000000000000, 0.000000000000000000 ) ) ;
#59084=CARTESIAN_POINT ( 'NONE',  ( 46.66904755831212981, 15.55634918610394379, 2.000000000000001776 ) ) ;
#59096=VECTOR ( 'NONE', #33945, 1000.000000000000000 ) ;
#59110=ORIENTED_EDGE ( 'NONE', *, *, #5876, .T. ) ;
#59125=CARTESIAN_POINT ( 'NONE',  ( 31.11269837220812562, 31.11269837220800483, 85.00100000000000477 ) ) ;
#59140=CARTESIAN_POINT ( 'NONE',  ( -51.66904755831212981, -10.55634918610397222, 0.000000000000000000 ) ) ;
#59142=EDGE_CURVE ( 'NONE', #8416, #65524, #58784, .T. ) ;
#59151=VERTEX_POINT ( 'NONE', #42949 ) ;
#59163=CARTESIAN_POINT ( 'NONE',  ( 0.000000000000000000, 0.000000000000000000, 17.57656211871651308 ) ) ;
#59170=CARTESIAN_POINT ( 'NONE',  ( -65.00000000000000000, 7.960204194457797252E-15, 15.70156211871650775 ) ) ;
#59178=VERTEX_POINT ( 'NONE', #39428 ) ;
#59209=LINE ( 'NONE', #53924, #41256 ) ;
#59220=ORIENTED_EDGE ( 'NONE', *, *, #2401, .F. ) ;
#59227=AXIS2_PLACEMENT_3D ( 'NONE', #51067, #45435, #13435 ) ;
#59237=CIRCLE ( 'NONE', #7607, 54.03875030502680943 ) ;
#59239=ADVANCED_FACE ( 'NONE', ( #23140 ), #1326, .F. ) ;
#59241=EDGE_CURVE ( 'NONE', #47843, #31978, #49847, .T. ) ;
#59242=VERTEX_POINT ( 'NONE', #984 ) ;
#59255=VECTOR ( 'NONE', #23259, 1000.000000000000000 ) ;
#59264=ORIENTED_EDGE ( 'NONE', *, *, #69308, .F. ) ;
#59267=VERTEX_POINT ( 'NONE', #34041 ) ;
#59268=ORIENTED_EDGE ( 'NONE', *, *, #54602, .F. ) ;
#59282=CARTESIAN_POINT ( 'NONE',  ( 0.000000000000000000, 0.000000000000000000, 26.24939009510892518 ) ) ;
#59285=APPLICATION_CONTEXT ( 'automotive_design' ) ;
#59347=CARTESIAN_POINT ( 'NONE',  ( -20.55634918610396866, 31.11269837220809009, 2.000000000000001776 ) ) ;
#59353=CARTESIAN_POINT ( 'NONE',  ( -31.11269837220804035, 15.55634918610408945, 2.000000000000001776 ) ) ;
#59370=CARTESIAN_POINT ( 'NONE',  ( -15.55634918610411077, -46.66904755831208718, 2.000000000000001776 ) ) ;
#59382=EDGE_CURVE ( 'NONE', #64323, #11967, #55438, .T. ) ;
#59389=EDGE_CURVE ( 'NONE', #46344, #50609, #7959, .T. ) ;
#59396=DIRECTION ( 'NONE',  ( -0.000000000000000000, -1.000000000000000000, -0.000000000000000000 ) ) ;
#59405=DIRECTION ( 'NONE',  ( 0.000000000000000000, 0.000000000000000000, -1.000000000000000000 ) ) ;
#59413=EDGE_LOOP ( 'NONE', ( #68196, #50294, #31845, #24164 ) ) ;
#59420=CARTESIAN_POINT ( 'NONE',  ( 26.11269837220812562, 36.11269837220800838, 2.000000000000001776 ) ) ;
#59455=ORIENTED_EDGE ( 'NONE', *, *, #55857, .T. ) ;
#59458=LINE ( 'NONE', #54526, #24488 ) ;
#59486=DIRECTION ( 'NONE',  ( 0.000000000000000000, -1.000000000000000000, 0.000000000000000000 ) ) ;
#59488=CARTESIAN_POINT ( 'NONE',  ( 15.55634918610409656, 36.11269837220803680, 0.000000000000000000 ) ) ;
#59510=PLANE ( 'NONE',  #46757 ) ;
#59515=LINE ( 'NONE', #32457, #51192 ) ;
#59524=ORIENTED_EDGE ( 'NONE', *, *, #23572, .F. ) ;
#59529=ORIENTED_EDGE ( 'NONE', *, *, #47087, .T. ) ;
#59531=EDGE_CURVE ( 'NONE', #7527, #19609, #1122, .T. ) ;
#59536=DIRECTION ( 'NONE',  ( -0.000000000000000000, -0.000000000000000000, -1.000000000000000000 ) ) ;
#59553=LINE ( 'NONE', #5060, #6324 ) ;
#59604=VERTEX_POINT ( 'NONE', #40148 ) ;
#59607=CARTESIAN_POINT ( 'NONE',  ( 0.000000000000000000, 0.000000000000000000, 25.00000000000007816 ) ) ;
#59618=ORIENTED_EDGE ( 'NONE', *, *, #60033, .F. ) ;
#59621=FACE_BOUND ( 'NONE', #20913, .T. ) ;
#59623=ADVANCED_FACE ( 'NONE', ( #46105 ), #51403, .F. ) ;
#59630=EDGE_CURVE ( 'NONE', #16162, #15169, #39800, .T. ) ;
#59631=ORIENTED_EDGE ( 'NONE', *, *, #42561, .T. ) ;
#59641=ORIENTED_EDGE ( 'NONE', *, *, #45169, .T. ) ;
#59654=ORIENTED_EDGE ( 'NONE', *, *, #45032, .F. ) ;
#59666=LINE ( 'NONE', #37886, #42753 ) ;
#59679=EDGE_LOOP ( 'NONE', ( #49366, #7492, #22441, #25120 ) ) ;
#59689=ADVANCED_FACE ( 'NONE', ( #56669 ), #49996, .F. ) ;
#59692=EDGE_CURVE ( 'NONE', #63697, #10376, #34541, .T. ) ;
#59710=CARTESIAN_POINT ( 'NONE',  ( 15.55634918610411610, 46.66904755831205875, 0.000000000000000000 ) ) ;
#59732=CARTESIAN_POINT ( 'NONE',  ( -15.55634918610411077, -46.66904755831208718, 0.000000000000000000 ) ) ;
#59758=AXIS2_PLACEMENT_3D ( 'NONE', #44299, #33766, #23217 ) ;
#59759=LINE ( 'NONE', #49553, #15938 ) ;
#59807=LINE ( 'NONE', #22189, #21060 ) ;
#59811=CARTESIAN_POINT ( 'NONE',  ( 10.55634918610406281, 15.55634918610400241, 2.000000000000001776 ) ) ;
#59833=DIRECTION ( 'NONE',  ( -0.000000000000000000, -0.000000000000000000, -1.000000000000000000 ) ) ;
#59845=DIRECTION ( 'NONE',  ( 0.000000000000000000, 1.000000000000000000, -0.000000000000000000 ) ) ;
#59865=DIRECTION ( 'NONE',  ( -0.000000000000000000, -1.000000000000000000, -0.000000000000000000 ) ) ;
#59869=DIRECTION ( 'NONE',  ( -0.000000000000000000, -0.000000000000000000, -1.000000000000000000 ) ) ;
#59872=ORIENTED_EDGE ( 'NONE', *, *, #52548, .F. ) ;
#59910=DIRECTION ( 'NONE',  ( -1.000000000000000000, 0.000000000000000000, 0.000000000000000000 ) ) ;
#59928=CARTESIAN_POINT ( 'NONE',  ( 15.55634918610411610, 46.66904755831205875, 2.000000000000001776 ) ) ;
#59940=DIRECTION ( 'NONE',  ( 1.000000000000000000, -0.000000000000000000, 0.000000000000000000 ) ) ;
#59952=LINE ( 'NONE', #1226, #52574 ) ;
#59960=VERTEX_POINT ( 'NONE', #49117 ) ;
#59962=AXIS2_PLACEMENT_3D ( 'NONE', #44584, #7302, #66064 ) ;
#59975=CARTESIAN_POINT ( 'NONE',  ( -2.645453300864630819E-14, -10.55634918610403439, 85.00100000000000477 ) ) ;
#59976=FACE_BOUND ( 'NONE', #66897, .T. ) ;
#59977=LINE ( 'NONE', #48715, #11310 ) ;
#59978=LINE ( 'NONE', #22358, #61242 ) ;
#59984=EDGE_CURVE ( 'NONE', #21979, #59267, #26985, .T. ) ;
#59993=LINE ( 'NONE', #39260, #45275 ) ;
#59995=ORIENTED_EDGE ( 'NONE', *, *, #12473, .F. ) ;
#60004=DIRECTION ( 'NONE',  ( -1.000000000000000000, 0.000000000000000000, 0.000000000000000000 ) ) ;
#60022=CARTESIAN_POINT ( 'NONE',  ( -20.55634918610396866, 31.11269837220809009, 85.00100000000000477 ) ) ;
#60028=PLANE ( 'NONE',  #52236 ) ;
#60030=DIRECTION ( 'NONE',  ( -0.000000000000000000, -0.000000000000000000, -1.000000000000000000 ) ) ;
#60033=EDGE_CURVE ( 'NONE', #32423, #34252, #49824, .T. ) ;
#60057=CARTESIAN_POINT ( 'NONE',  ( -31.11269837220806878, 5.000000000000056843, 0.000000000000000000 ) ) ;
#60069=EDGE_LOOP ( 'NONE', ( #63297, #25306, #40599, #64712 ) ) ;
#60088=DIRECTION ( 'NONE',  ( -1.000000000000000000, 0.000000000000000000, 0.000000000000000000 ) ) ;
#60095=CARTESIAN_POINT ( 'NONE',  ( -7.329206686002009974E-14, -46.66904755831211560, 0.000000000000000000 ) ) ;
#60109=DIRECTION ( 'NONE',  ( -0.000000000000000000, -0.000000000000000000, -1.000000000000000000 ) ) ;
#60146=CARTESIAN_POINT ( 'NONE',  ( -36.11269837220812207, -31.11269837220801193, 85.00100000000000477 ) ) ;
#60148=LINE ( 'NONE', #33440, #21644 ) ;
#60150=VECTOR ( 'NONE', #35013, 1000.000000000000000 ) ;
#60156=LINE ( 'NONE', #16894, #47409 ) ;
#60185=EDGE_CURVE ( 'NONE', #42033, #14102, #56496, .T. ) ;
#60190=FACE_OUTER_BOUND ( 'NONE', #22499, .T. ) ;
#60217=LINE ( 'NONE', #11322, #45312 ) ;
#60228=DIRECTION ( 'NONE',  ( 1.000000000000000000, 0.000000000000000000, 0.000000000000000000 ) ) ;
#60263=ORIENTED_EDGE ( 'NONE', *, *, #51380, .T. ) ;
#60270=LINE ( 'NONE', #14745, #1335 ) ;
#60272=EDGE_CURVE ( 'NONE', #24929, #38551, #37115, .T. ) ;
#60283=CARTESIAN_POINT ( 'NONE',  ( -4.999999999999971578, 20.55634918610402906, 85.00100000000000477 ) ) ;
#60284=FILL_AREA_STYLE ('',( #12097 ) ) ;
#60290=VERTEX_POINT ( 'NONE', #48001 ) ;
#60291=EDGE_LOOP ( 'NONE', ( #50145, #15647, #607, #49702 ) ) ;
#60316=EDGE_LOOP ( 'NONE', ( #3541, #56962, #45994, #43851 ) ) ;
#60317=VECTOR ( 'NONE', #19481, 1000.000000000000000 ) ;
#60322=ORIENTED_EDGE ( 'NONE', *, *, #53111, .T. ) ;
#60333=EDGE_CURVE ( 'NONE', #43731, #44813, #16693, .T. ) ;
#60336=ORIENTED_EDGE ( 'NONE', *, *, #47340, .F. ) ;
#60348=VECTOR ( 'NONE', #37914, 1000.000000000000000 ) ;
#60373=DIRECTION ( 'NONE',  ( 1.000000000000000000, -0.000000000000000000, 0.000000000000000000 ) ) ;
#60392=FACE_OUTER_BOUND ( 'NONE', #62432, .T. ) ;
#60397=ORIENTED_EDGE ( 'NONE', *, *, #12819, .T. ) ;
#60418=CARTESIAN_POINT ( 'NONE',  ( -15.55634918610400597, 15.55634918610405748, 85.00100000000000477 ) ) ;
#60427=DIRECTION ( 'NONE',  ( -0.000000000000000000, -1.000000000000000000, -0.000000000000000000 ) ) ;
#60456=VECTOR ( 'NONE', #59865, 1000.000000000000000 ) ;
#60460=FACE_OUTER_BOUND ( 'NONE', #5967, .T. ) ;
#60470=ORIENTED_EDGE ( 'NONE', *, *, #790, .T. ) ;
#60496=CARTESIAN_POINT ( 'NONE',  ( 0.000000000000000000, 0.000000000000000000, 26.24939009510892518 ) ) ;
#60504=ORIENTED_EDGE ( 'NONE', *, *, #32565, .T. ) ;
#60524=DIRECTION ( 'NONE',  ( 0.000000000000000000, 0.000000000000000000, 1.000000000000000000 ) ) ;
#60541=ORIENTED_EDGE ( 'NONE', *, *, #4123, .T. ) ;
#60544=CARTESIAN_POINT ( 'NONE',  ( 26.11269837220803325, -15.55634918610409656, 2.000000000000001776 ) ) ;
#60549=CARTESIAN_POINT ( 'NONE',  ( -15.55634918610408945, -31.11269837220804035, 2.000000000000001776 ) ) ;
#60552=VERTEX_POINT ( 'NONE', #13853 ) ;
#60572=VERTEX_POINT ( 'NONE', #56772 ) ;
#60600=DIRECTION ( 'NONE',  ( -0.000000000000000000, -0.000000000000000000, -1.000000000000000000 ) ) ;
#60612=VECTOR ( 'NONE', #47246, 1000.000000000000000 ) ;
#60657=ADVANCED_FACE ( 'NONE', ( #5704 ), #41969, .F. ) ;
#60675=PLANE ( 'NONE',  #12211 ) ;
#60678=ADVANCED_FACE ( 'NONE', ( #69388 ), #59510, .F. ) ;
#60679=CARTESIAN_POINT ( 'NONE',  ( 0.000000000000000000, 0.000000000000000000, 85.00000000000000000 ) ) ;
#60683=CARTESIAN_POINT ( 'NONE',  ( -5.000000000000058620, -26.11269837220806522, 0.000000000000000000 ) ) ;
#60708=DIRECTION ( 'NONE',  ( -0.000000000000000000, -0.000000000000000000, -1.000000000000000000 ) ) ;
#60716=PLANE ( 'NONE',  #68858 ) ;
#60723=LINE ( 'NONE', #61757, #38938 ) ;
#60724=DIRECTION ( 'NONE',  ( 0.000000000000000000, 1.000000000000000000, -0.000000000000000000 ) ) ;
#60744=DIRECTION ( 'NONE',  ( -0.000000000000000000, -0.000000000000000000, -1.000000000000000000 ) ) ;
#60747=EDGE_LOOP ( 'NONE', ( #18678, #41365, #12867, #36404 ) ) ;
#60758=CARTESIAN_POINT ( 'NONE',  ( 15.55634918610397399, -31.11269837220809364, 0.000000000000000000 ) ) ;
#60771=FACE_BOUND ( 'NONE', #17932, .T. ) ;
#60808=ORIENTED_EDGE ( 'NONE', *, *, #41454, .F. ) ;
#60815=EDGE_CURVE ( 'NONE', #63697, #33686, #45661, .T. ) ;
#60822=VECTOR ( 'NONE', #38503, 1000.000000000000000 ) ;
#60844=AXIS2_PLACEMENT_3D ( 'NONE', #41176, #41865, #9860 ) ;
#60856=LINE ( 'NONE', #371, #32305 ) ;
#60873=EDGE_CURVE ( 'NONE', #58260, #62528, #62574, .T. ) ;
#60884=CYLINDRICAL_SURFACE ( 'NONE', #7106, 72.99999999999998579 ) ;
#60903=PLANE ( 'NONE',  #52091 ) ;
#60927=AXIS2_PLACEMENT_3D ( 'NONE', #68482, #9398, #30855 ) ;
#60938=VERTEX_POINT ( 'NONE', #5878 ) ;
#60939=VECTOR ( 'NONE', #36548, 1000.000000000000000 ) ;
#60982=ORIENTED_EDGE ( 'NONE', *, *, #5444, .F. ) ;
#60983=ORIENTED_EDGE ( 'NONE', *, *, #16012, .F. ) ;
#60992=VECTOR ( 'NONE', #63133, 1000.000000000000000 ) ;
#61045=FACE_OUTER_BOUND ( 'NONE', #53303, .T. ) ;
#61056=VERTEX_POINT ( 'NONE', #57555 ) ;
#61065=VERTEX_POINT ( 'NONE', #15333 ) ;
#61075=CARTESIAN_POINT ( 'NONE',  ( 10.55634918610400419, -15.55634918610406103, 2.000000000000001776 ) ) ;
#61084=ORIENTED_EDGE ( 'NONE', *, *, #64555, .F. ) ;
#61118=ORIENTED_EDGE ( 'NONE', *, *, #44854, .T. ) ;
#61133=VECTOR ( 'NONE', #40261, 1000.000000000000000 ) ;
#61165=ORIENTED_EDGE ( 'NONE', *, *, #17807, .F. ) ;
#61172=ORIENTED_EDGE ( 'NONE', *, *, #3482, .T. ) ;
#61181=ORIENTED_EDGE ( 'NONE', *, *, #32554, .F. ) ;
#61183=LINE ( 'NONE', #43937, #47300 ) ;
#61227=EDGE_CURVE ( 'NONE', #63672, #59242, #17763, .T. ) ;
#61242=VECTOR ( 'NONE', #557, 1000.000000000000000 ) ;
#61258=CARTESIAN_POINT ( 'NONE',  ( -20.55634918610408945, -31.11269837220804035, 85.00100000000000477 ) ) ;
#61270=VERTEX_POINT ( 'NONE', #13528 ) ;
#61330=DIRECTION ( 'NONE',  ( 0.000000000000000000, -1.000000000000000000, 0.000000000000000000 ) ) ;
#61369=CARTESIAN_POINT ( 'NONE',  ( -7.329206686002009974E-14, -41.66904755831212270, 85.00100000000000477 ) ) ;
#61370=ORIENTED_EDGE ( 'NONE', *, *, #51926, .T. ) ;
#61418=ORIENTED_EDGE ( 'NONE', *, *, #47687, .T. ) ;
#61446=FACE_OUTER_BOUND ( 'NONE', #9437, .T. ) ;
#61451=LINE ( 'NONE', #34731, #48186 ) ;
#61464=EDGE_CURVE ( 'NONE', #10168, #8516, #13861, .T. ) ;
#61466=ADVANCED_FACE ( 'NONE', ( #41976 ), #14893, .F. ) ;
#61467=ORIENTED_EDGE ( 'NONE', *, *, #48585, .T. ) ;
#61492=EDGE_CURVE ( 'NONE', #1617, #63246, #68376, .T. ) ;
#61497=EDGE_CURVE ( 'NONE', #13782, #63246, #67347, .T. ) ;
#61505=ORIENTED_EDGE ( 'NONE', *, *, #36076, .T. ) ;
#61521=PLANE ( 'NONE',  #19902 ) ;
#61533=LINE ( 'NONE', #39380, #15874 ) ;
#61539=CARTESIAN_POINT ( 'NONE',  ( -36.11269837220809364, -10.55634918610397932, 0.000000000000000000 ) ) ;
#61586=PLANE ( 'NONE',  #31019 ) ;
#61588=ORIENTED_EDGE ( 'NONE', *, *, #68411, .T. ) ;
#61590=CARTESIAN_POINT ( 'NONE',  ( 0.000000000000000000, 0.000000000000000000, 85.00000000000000000 ) ) ;
#61592=LINE ( 'NONE', #32206, #39738 ) ;
#61593=CARTESIAN_POINT ( 'NONE',  ( 6.375108774214766072E-14, 36.11269837220805812, 0.000000000000000000 ) ) ;
#61604=DIRECTION ( 'NONE',  ( -0.000000000000000000, -0.000000000000000000, -1.000000000000000000 ) ) ;
#61606=DIRECTION ( 'NONE',  ( 0.000000000000000000, 1.000000000000000000, -0.000000000000000000 ) ) ;
#61615=EDGE_CURVE ( 'NONE', #38817, #57581, #44757, .T. ) ;
#61649=EDGE_LOOP ( 'NONE', ( #5669, #26315 ) ) ;
#61701=FACE_OUTER_BOUND ( 'NONE', #11732, .T. ) ;
#61712=ORIENTED_EDGE ( 'NONE', *, *, #11245, .F. ) ;
#61722=DIRECTION ( 'NONE',  ( -0.000000000000000000, -0.000000000000000000, -1.000000000000000000 ) ) ;
#61730=EDGE_LOOP ( 'NONE', ( #30660, #63824, #26454, #27755 ) ) ;
#61742=CARTESIAN_POINT ( 'NONE',  ( 41.66904755831208007, -15.55634918610412853, 0.000000000000000000 ) ) ;
#61743=VECTOR ( 'NONE', #13315, 1000.000000000000000 ) ;
#61747=CARTESIAN_POINT ( 'NONE',  ( 31.11269837220800127, -26.11269837220812562, 2.000000000000001776 ) ) ;
#61748=DIRECTION ( 'NONE',  ( -1.000000000000000000, 0.000000000000000000, 0.000000000000000000 ) ) ;
#61753=DIRECTION ( 'NONE',  ( 1.000000000000000000, -0.000000000000000000, -0.000000000000000000 ) ) ;
#61757=CARTESIAN_POINT ( 'NONE',  ( -15.55634918610405748, -15.55634918610400774, 0.000000000000000000 ) ) ;
#61784=ADVANCED_BREP_SHAPE_REPRESENTATION ( '', ( #16293, #66832 ), #51149 ) ;
#61786=CARTESIAN_POINT ( 'NONE',  ( 0.000000000000000000, 0.000000000000000000, 85.00000000000000000 ) ) ;
#61820=DIRECTION ( 'NONE',  ( 0.000000000000000000, 0.000000000000000000, 1.000000000000000000 ) ) ;
#61821=CARTESIAN_POINT ( 'NONE',  ( -31.11269837220806878, 5.000000000000056843, 0.000000000000000000 ) ) ;
#61923=CARTESIAN_POINT ( 'NONE',  ( -5.767955557622883589E-14, -31.11269837220806878, 0.000000000000000000 ) ) ;
#61924=CIRCLE ( 'NONE', #43938, 65.00000000000000000 ) ;
#61941=AXIS2_PLACEMENT_3D ( 'NONE', #57353, #62971, #51727 ) ;
#61973=PLANE ( 'NONE',  #19138 ) ;
#61975=AXIS2_PLACEMENT_3D ( 'NONE', #40863, #39824, #56696 ) ;
#61988=EDGE_LOOP ( 'NONE', ( #59268, #11977 ) ) ;
#61991=CARTESIAN_POINT ( 'NONE',  ( 7.762887554996211747E-14, 46.66904755831208718, 85.00100000000000477 ) ) ;
#62001=EDGE_CURVE ( 'NONE', #61270, #8605, #22693, .T. ) ;
#62027=VERTEX_POINT ( 'NONE', #18123 ) ;
#62041=CARTESIAN_POINT ( 'NONE',  ( -2.645453300864630819E-14, -10.55634918610403439, 0.000000000000000000 ) ) ;
#62046=ORIENTED_EDGE ( 'NONE', *, *, #30585, .T. ) ;
#62070=ORIENTED_EDGE ( 'NONE', *, *, #47261, .T. ) ;
#62074=EDGE_CURVE ( 'NONE', #35107, #46320, #67125, .T. ) ;
#62086=EDGE_CURVE ( 'NONE', #17852, #11222, #18812, .T. ) ;
#62089=ORIENTED_EDGE ( 'NONE', *, *, #64291, .F. ) ;
#62093=CARTESIAN_POINT ( 'NONE',  ( -15.55634918610405748, -10.55634918610400597, 2.000000000000001776 ) ) ;
#62101=EDGE_LOOP ( 'NONE', ( #40092, #4532, #50345, #21310 ) ) ;
#62105=EDGE_CURVE ( 'NONE', #55128, #61056, #9290, .T. ) ;
#62135=DIRECTION ( 'NONE',  ( 1.000000000000000000, 0.000000000000000000, 0.000000000000000000 ) ) ;
#62136=VERTEX_POINT ( 'NONE', #52202 ) ;
#62157=FACE_BOUND ( 'NONE', #33563, .T. ) ;
#62189=DIRECTION ( 'NONE',  ( 0.000000000000000000, 0.000000000000000000, 1.000000000000000000 ) ) ;
#62199=DIRECTION ( 'NONE',  ( 1.000000000000000000, -0.000000000000000000, 0.000000000000000000 ) ) ;
#62228=ORIENTED_EDGE ( 'NONE', *, *, #30475, .T. ) ;
#62230=VECTOR ( 'NONE', #21097, 1000.000000000000000 ) ;
#62274=ADVANCED_FACE ( 'NONE', ( #54247 ), #32127, .F. ) ;
#62292=LINE ( 'NONE', #8489, #8613 ) ;
#62300=ORIENTED_EDGE ( 'NONE', *, *, #15982, .F. ) ;
#62306=ORIENTED_EDGE ( 'NONE', *, *, #11245, .T. ) ;
#62320=VECTOR ( 'NONE', #1346, 1000.000000000000000 ) ;
#62324=VECTOR ( 'NONE', #65891, 1000.000000000000000 ) ;
#62340=DIRECTION ( 'NONE',  ( 0.000000000000000000, 0.000000000000000000, 1.000000000000000000 ) ) ;
#62349=LINE ( 'NONE', #26445, #50648 ) ;
#62356=CARTESIAN_POINT ( 'NONE',  ( 31.11269837220812562, 36.11269837220800838, 85.00100000000000477 ) ) ;
#62358=EDGE_LOOP ( 'NONE', ( #46067, #12647, #59618, #46232 ) ) ;
#62373=EDGE_CURVE ( 'NONE', #43813, #54143, #53048, .T. ) ;
#62376=EDGE_LOOP ( 'NONE', ( #40899, #26632, #4433, #34017 ) ) ;
#62378=CARTESIAN_POINT ( 'NONE',  ( 10.55634918610397577, -26.11269837220809364, 2.000000000000001776 ) ) ;
#62387=PLANE ( 'NONE',  #31548 ) ;
#62393=AXIS2_PLACEMENT_3D ( 'NONE', #58771, #37669, #32057 ) ;
#62429=EDGE_CURVE ( 'NONE', #62781, #43813, #6254, .T. ) ;
#62431=FACE_OUTER_BOUND ( 'NONE', #5243, .T. ) ;
#62432=EDGE_LOOP ( 'NONE', ( #40905, #27758, #68750, #14273 ) ) ;
#62437=CARTESIAN_POINT ( 'NONE',  ( 15.55634918610406103, 20.55634918610400064, 85.00100000000000477 ) ) ;
#62439=CARTESIAN_POINT ( 'NONE',  ( 15.55634918610396511, -46.66904755831214402, 2.000000000000001776 ) ) ;
#62441=CARTESIAN_POINT ( 'NONE',  ( -46.66904755831210139, 5.000000000000066613, 85.00100000000000477 ) ) ;
#62442=LINE ( 'NONE', #19172, #44405 ) ;
#62445=AXIS2_PLACEMENT_3D ( 'NONE', #20740, #37820, #21421 ) ;
#62463=CARTESIAN_POINT ( 'NONE',  ( -4.999999999999922728, 46.66904755831208718, 85.00100000000000477 ) ) ;
#62464=LINE ( 'NONE', #56143, #62630 ) ;
#62479=VECTOR ( 'NONE', #58979, 1000.000000000000000 ) ;
#62516=ADVANCED_FACE ( 'NONE', ( #1248 ), #34534, .F. ) ;
#62528=VERTEX_POINT ( 'NONE', #27626 ) ;
#62543=ORIENTED_EDGE ( 'NONE', *, *, #16669, .T. ) ;
#62564=DIRECTION ( 'NONE',  ( 0.000000000000000000, 0.000000000000000000, 1.000000000000000000 ) ) ;
#62574=LINE ( 'NONE', #30219, #31059 ) ;
#62593=AXIS2_PLACEMENT_3D ( 'NONE', #455, #42675, #5395 ) ;
#62602=ADVANCED_FACE ( 'NONE', ( #22008 ), #16720, .F. ) ;
#62608=ORIENTED_EDGE ( 'NONE', *, *, #57745, .T. ) ;
#62623=DIRECTION ( 'NONE',  ( 1.000000000000000000, -0.000000000000000000, 0.000000000000000000 ) ) ;
#62630=VECTOR ( 'NONE', #57191, 1000.000000000000000 ) ;
#62635=VECTOR ( 'NONE', #54489, 1000.000000000000000 ) ;
#62636=FACE_OUTER_BOUND ( 'NONE', #52585, .T. ) ;
#62652=CARTESIAN_POINT ( 'NONE',  ( 0.000000000000000000, 5.000000000000000000, 0.000000000000000000 ) ) ;
#62661=ADVANCED_FACE ( 'NONE', ( #16386 ), #904, .F. ) ;
#62672=ORIENTED_EDGE ( 'NONE', *, *, #53812, .T. ) ;
#62681=EDGE_CURVE ( 'NONE', #40853, #43873, #19159, .T. ) ;
#62692=VECTOR ( 'NONE', #45408, 999.9999999999998863 ) ;
#62697=CARTESIAN_POINT ( 'NONE',  ( -5.000000000000000000, 0.000000000000000000, 0.000000000000000000 ) ) ;
#62700=LINE ( 'NONE', #53142, #16271 ) ;
#62703=DIRECTION ( 'NONE',  ( 0.000000000000000000, 0.000000000000000000, 1.000000000000000000 ) ) ;
#62726=VERTEX_POINT ( 'NONE', #30075 ) ;
#62749=CARTESIAN_POINT ( 'NONE',  ( 7.762887554996211747E-14, 51.66904755831208718, 0.000000000000000000 ) ) ;
#62759=DIRECTION ( 'NONE',  ( -1.000000000000000000, 0.000000000000000000, 0.000000000000000000 ) ) ;
#62768=ADVANCED_FACE ( 'NONE', ( #56106 ), #2645, .F. ) ;
#62781=VERTEX_POINT ( 'NONE', #52550 ) ;
#62782=VECTOR ( 'NONE', #18624, 1000.000000000000000 ) ;
#62803=ORIENTED_EDGE ( 'NONE', *, *, #6103, .F. ) ;
#62805=VERTEX_POINT ( 'NONE', #14913 ) ;
#62821=DIRECTION ( 'NONE',  ( -0.000000000000000000, -1.000000000000000000, -0.000000000000000000 ) ) ;
#62836=EDGE_CURVE ( 'NONE', #29447, #51672, #68721, .T. ) ;
#62839=ORIENTED_EDGE ( 'NONE', *, *, #14314, .F. ) ;
#62876=DIRECTION ( 'NONE',  ( 0.000000000000000000, 1.000000000000000000, 0.000000000000000000 ) ) ;
#62899=EDGE_LOOP ( 'NONE', ( #62938, #65835, #7791, #15780 ) ) ;
#62926=VERTEX_POINT ( 'NONE', #8182 ) ;
#62932=VERTEX_POINT ( 'NONE', #24715 ) ;
#62934=ORIENTED_EDGE ( 'NONE', *, *, #16192, .F. ) ;
#62938=ORIENTED_EDGE ( 'NONE', *, *, #5300, .F. ) ;
#62940=VECTOR ( 'NONE', #51889, 1000.000000000000000 ) ;
#62954=VECTOR ( 'NONE', #27748, 1000.000000000000000 ) ;
#62963=EDGE_CURVE ( 'NONE', #30890, #37055, #13460, .T. ) ;
#62971=DIRECTION ( 'NONE',  ( -1.000000000000000000, 0.000000000000000000, 0.000000000000000000 ) ) ;
#62993=VECTOR ( 'NONE', #2449, 1000.000000000000000 ) ;
#63008=ORIENTED_EDGE ( 'NONE', *, *, #14702, .F. ) ;
#63009=LINE ( 'NONE', #20102, #29192 ) ;
#63071=PLANE ( 'NONE',  #51390 ) ;
#63078=LINE ( 'NONE', #41623, #18355 ) ;
#63083=DIRECTION ( 'NONE',  ( 0.000000000000000000, 1.000000000000000000, -0.000000000000000000 ) ) ;
#63085=CARTESIAN_POINT ( 'NONE',  ( 41.66904755831210849, -9.150666335777657423E-14, 0.000000000000000000 ) ) ;
#63090=VECTOR ( 'NONE', #51077, 1000.000000000000000 ) ;
#63091=ORIENTED_EDGE ( 'NONE', *, *, #59984, .F. ) ;
#63100=PLANE ( 'NONE',  #49336 ) ;
#63127=EDGE_CURVE ( 'NONE', #31978, #24127, #64396, .T. ) ;
#63133=DIRECTION ( 'NONE',  ( -0.000000000000000000, -1.000000000000000000, -0.000000000000000000 ) ) ;
#63136=EDGE_CURVE ( 'NONE', #22403, #56265, #59458, .T. ) ;
#63145=LINE ( 'NONE', #35729, #9039 ) ;
#63155=EDGE_CURVE ( 'NONE', #53816, #46344, #43970, .T. ) ;
#63161=LINE ( 'NONE', #2426, #24046 ) ;
#63167=DIRECTION ( 'NONE',  ( 0.000000000000000000, 1.000000000000000000, -0.000000000000000000 ) ) ;
#63240=VECTOR ( 'NONE', #52150, 1000.000000000000000 ) ;
#63246=VERTEX_POINT ( 'NONE', #23588 ) ;
#63287=EDGE_LOOP ( 'NONE', ( #62070, #27113, #12963, #67602 ) ) ;
#63297=ORIENTED_EDGE ( 'NONE', *, *, #36948, .T. ) ;
#63308=CARTESIAN_POINT ( 'NONE',  ( 15.55634918610403261, -3.079134169858832593E-14, 0.000000000000000000 ) ) ;
#63322=DIRECTION ( 'NONE',  ( -0.000000000000000000, -0.000000000000000000, -1.000000000000000000 ) ) ;
#63323=CARTESIAN_POINT ( 'NONE',  ( 46.66904755831212981, 15.55634918610394379, 0.000000000000000000 ) ) ;
#63328=FACE_OUTER_BOUND ( 'NONE', #7332, .T. ) ;
#63347=ORIENTED_EDGE ( 'NONE', *, *, #47237, .T. ) ;
#63361=EDGE_CURVE ( 'NONE', #52273, #62726, #204, .T. ) ;
#63366=EDGE_CURVE ( 'NONE', #51103, #44250, #24978, .T. ) ;
#63382=EDGE_CURVE ( 'NONE', #19486, #22868, #565, .T. ) ;
#63405=ORIENTED_EDGE ( 'NONE', *, *, #37873, .T. ) ;
#63413=DIRECTION ( 'NONE',  ( 1.000000000000000000, -0.000000000000000000, -0.000000000000000000 ) ) ;
#63420=DIRECTION ( 'NONE',  ( -0.000000000000000000, -1.000000000000000000, -0.000000000000000000 ) ) ;
#63432=ORIENTED_EDGE ( 'NONE', *, *, #59142, .F. ) ;
#63439=VECTOR ( 'NONE', #62821, 1000.000000000000000 ) ;
#63466=DIRECTION ( 'NONE',  ( -0.6246950475544236214, 7.650307904307285654E-17, 0.7808688094430308313 ) ) ;
#63469=ORIENTED_EDGE ( 'NONE', *, *, #39057, .T. ) ;
#63493=VECTOR ( 'NONE', #53909, 1000.000000000000000 ) ;
#63497=DIRECTION ( 'NONE',  ( 0.000000000000000000, 0.000000000000000000, 1.000000000000000000 ) ) ;
#63503=CARTESIAN_POINT ( 'NONE',  ( 31.11269837220800127, -26.11269837220812562, 2.000000000000001776 ) ) ;
#63511=ORIENTED_EDGE ( 'NONE', *, *, #9597, .T. ) ;
#63531=CARTESIAN_POINT ( 'NONE',  ( -31.11269837220812207, -26.11269837220801193, 2.000000000000001776 ) ) ;
#63532=ADVANCED_FACE ( 'NONE', ( #61045 ), #35710, .F. ) ;
#63538=ORIENTED_EDGE ( 'NONE', *, *, #26354, .T. ) ;
#63548=CARTESIAN_POINT ( 'NONE',  ( 10.55634918610411432, 46.66904755831205875, 2.000000000000000000 ) ) ;
#63549=EDGE_LOOP ( 'NONE', ( #60397, #32980, #39445, #10574 ) ) ;
#63618=LINE ( 'NONE', #47417, #18783 ) ;
#63634=VERTEX_POINT ( 'NONE', #69428 ) ;
#63656=DIRECTION ( 'NONE',  ( -0.000000000000000000, -1.000000000000000000, -0.000000000000000000 ) ) ;
#63672=VERTEX_POINT ( 'NONE', #64501 ) ;
#63689=CARTESIAN_POINT ( 'NONE',  ( 31.11269837220806522, 0.000000000000000000, 0.000000000000000000 ) ) ;
#63697=VERTEX_POINT ( 'NONE', #17712 ) ;
#63700=LINE ( 'NONE', #15510, #22182 ) ;
#63732=VECTOR ( 'NONE', #46925, 1000.000000000000000 ) ;
#63770=DIRECTION ( 'NONE',  ( 0.000000000000000000, 1.000000000000000000, -0.000000000000000000 ) ) ;
#63777=DIRECTION ( 'NONE',  ( 0.000000000000000000, -0.000000000000000000, -1.000000000000000000 ) ) ;
#63785=DIRECTION ( 'NONE',  ( 0.000000000000000000, -1.000000000000000000, 0.000000000000000000 ) ) ;
#63786=PLANE ( 'NONE',  #41097 ) ;
#63796=DIRECTION ( 'NONE',  ( 1.000000000000000000, -0.000000000000000000, 0.000000000000000000 ) ) ;
#63810=DIRECTION ( 'NONE',  ( 0.000000000000000000, -0.000000000000000000, -1.000000000000000000 ) ) ;
#63812=ORIENTED_EDGE ( 'NONE', *, *, #23350, .T. ) ;
#63824=ORIENTED_EDGE ( 'NONE', *, *, #54686, .T. ) ;
#63845=ADVANCED_FACE ( 'NONE', ( #58776 ), #16911, .F. ) ;
#63857=DIRECTION ( 'NONE',  ( -0.000000000000000000, -1.000000000000000000, -0.000000000000000000 ) ) ;
#63884=ORIENTED_EDGE ( 'NONE', *, *, #31692, .T. ) ;
#63899=DIRECTION ( 'NONE',  ( 0.000000000000000000, -1.000000000000000000, 0.000000000000000000 ) ) ;
#63903=LINE ( 'NONE', #64597, #12496 ) ;
#63914=EDGE_CURVE ( 'NONE', #65364, #7527, #50669, .T. ) ;
#63921=VECTOR ( 'NONE', #65178, 1000.000000000000000 ) ;
#63929=FACE_OUTER_BOUND ( 'NONE', #43454, .T. ) ;
#63934=FACE_OUTER_BOUND ( 'NONE', #54076, .T. ) ;
#63955=DIRECTION ( 'NONE',  ( 0.000000000000000000, 0.000000000000000000, 1.000000000000000000 ) ) ;
#63964=CARTESIAN_POINT ( 'NONE',  ( 2.905661822261151883E-14, 15.55634918610403084, 0.000000000000000000 ) ) ;
#63965=AXIS2_PLACEMENT_3D ( 'NONE', #19774, #62340, #57068 ) ;
#63981=ORIENTED_EDGE ( 'NONE', *, *, #25925, .F. ) ;
#63993=EDGE_CURVE ( 'NONE', #18531, #19486, #20735, .T. ) ;
#64009=ORIENTED_EDGE ( 'NONE', *, *, #63366, .F. ) ;
#64016=LINE ( 'NONE', #38576, #25578 ) ;
#64023=ADVANCED_FACE ( 'NONE', ( #300 ), #48817, .F. ) ;
#64030=PLANE ( 'NONE',  #65511 ) ;
#64031=LINE ( 'NONE', #59084, #41444 ) ;
#64033=ORIENTED_EDGE ( 'NONE', *, *, #54565, .F. ) ;
#64036=LINE ( 'NONE', #31680, #45102 ) ;
#64042=EDGE_LOOP ( 'NONE', ( #25013, #42254, #47960, #4161 ) ) ;
#64045=DIRECTION ( 'NONE',  ( 0.000000000000000000, 1.000000000000000000, -0.000000000000000000 ) ) ;
#64058=CARTESIAN_POINT ( 'NONE',  ( -20.55634918610403261, 2.818925648462311528E-14, 2.000000000000001776 ) ) ;
#64071=CARTESIAN_POINT ( 'NONE',  ( -5.767955557622883589E-14, -31.11269837220806878, 85.00100000000000477 ) ) ;
#64102=ORIENTED_EDGE ( 'NONE', *, *, #25292, .T. ) ;
#64114=ORIENTED_EDGE ( 'NONE', *, *, #10872, .T. ) ;
#64131=VECTOR ( 'NONE', #25092, 1000.000000000000000 ) ;
#64142=DIRECTION ( 'NONE',  ( -0.000000000000000000, -1.000000000000000000, -0.000000000000000000 ) ) ;
#64158=CARTESIAN_POINT ( 'NONE',  ( -46.66904755831212981, -15.55634918610397222, 2.000000000000001776 ) ) ;
#64201=VERTEX_POINT ( 'NONE', #18577 ) ;
#64205=EDGE_LOOP ( 'NONE', ( #59220, #62228, #46078, #25563 ) ) ;
#64222=FACE_BOUND ( 'NONE', #5264, .T. ) ;
#64247=CLOSED_SHELL ( 'NONE', ( #16018, #34904, #7311, #67619, #12082, #33439, #62516, #55257, #34559, #33853, #20557, #32270, #1249, #33205, #41718, #12883, #41225, #10303, #52800, #59039, #29955, #22942, #59239, #53685, #2865, #28693, #10394, #25324, #31074, #3093, #60657, #1759, #29687, #52435, #30645, #20447, #32797, #22202, #25983, #66553, #57975, #10624, #68972, #3747, #37414, #19294, #8344, #31289, #48042, #556, #7401, #64713, #10544, #46392, #50422, #39632, #36561, #69387, #21268, #63845, #2540, #32409, #41414, #39243, #57562, #38415, #28730, #60678, #62602, #66958, #13282, #62274, #22786, #66645, #61466, #12019, #54963, #51908, #7079, #2860, #63532, #27171, #30881, #59623, #18569, #16735, #64023, #8218, #17478, #20875, #47599, #27571, #30136, #20756, #19148, #34644, #49034, #40027, #6520, #62661, #32523, #39452, #40964, #8987, #10708, #9863, #57520, #49313, #21076, #20629, #62768, #18248, #69444, #4279, #17472, #45898, #18025, #20630, #3178, #58502, #58995, #20025, #322, #36214, #22451, #26744, #51178, #25118, #55442, #47646, #55249, #28037, #19532, #16420, #44880, #23822, #33691, #52243, #57891, #34863, #58994, #14117, #11900, #16680, #5547, #58343, #23138, #59689, #20578, #44305, #23824, #40815, #8213, #28166, #35700, #48971, #6676, #38158 ) ) ;
#64250=FACE_OUTER_BOUND ( 'NONE', #40060, .T. ) ;
#64266=LINE ( 'NONE', #69532, #27762 ) ;
#64267=DIRECTION ( 'NONE',  ( 0.000000000000000000, 1.000000000000000000, -0.000000000000000000 ) ) ;
#64274=CARTESIAN_POINT ( 'NONE',  ( 2.905661822261151883E-14, 15.55634918610403084, 2.000000000000001776 ) ) ;
#64291=EDGE_CURVE ( 'NONE', #33219, #69014, #64031, .T. ) ;
#64294=VECTOR ( 'NONE', #3465, 1000.000000000000000 ) ;
#64306=EDGE_CURVE ( 'NONE', #37055, #38069, #1053, .T. ) ;
#64309=LINE ( 'NONE', #42166, #43235 ) ;
#64323=VERTEX_POINT ( 'NONE', #26745 ) ;
#64335=ORIENTED_EDGE ( 'NONE', *, *, #56885, .T. ) ;
#64368=ORIENTED_EDGE ( 'NONE', *, *, #1192, .F. ) ;
#64370=LINE ( 'NONE', #16187, #45747 ) ;
#64371=LINE ( 'NONE', #32031, #68697 ) ;
#64396=LINE ( 'NONE', #1079, #66016 ) ;
#64405=VERTEX_POINT ( 'NONE', #13014 ) ;
#64407=EDGE_CURVE ( 'NONE', #57934, #8504, #49924, .T. ) ;
#64408=CARTESIAN_POINT ( 'NONE',  ( -36.11269837220809364, -15.55634918610397754, 0.000000000000000000 ) ) ;
#64437=VECTOR ( 'NONE', #43211, 1000.000000000000000 ) ;
#64438=EDGE_LOOP ( 'NONE', ( #43113, #19404, #69508, #21148 ) ) ;
#64462=LINE ( 'NONE', #16273, #48886 ) ;
#64470=ORIENTED_EDGE ( 'NONE', *, *, #64616, .T. ) ;
#64484=AXIS2_PLACEMENT_3D ( 'NONE', #8308, #20571, #35040 ) ;
#64490=VECTOR ( 'NONE', #20352, 1000.000000000000000 ) ;
#64498=EDGE_CURVE ( 'NONE', #29482, #63672, #40418, .T. ) ;
#64501=CARTESIAN_POINT ( 'NONE',  ( -5.000000000000073719, -46.66904755831211560, 0.000000000000000000 ) ) ;
#64503=FACE_OUTER_BOUND ( 'NONE', #65512, .T. ) ;
#64515=LINE ( 'NONE', #27217, #40607 ) ;
#64524=VECTOR ( 'NONE', #69499, 1000.000000000000000 ) ;
#64528=CARTESIAN_POINT ( 'NONE',  ( -2.645453300864630819E-14, -10.55634918610403439, 2.000000000000001776 ) ) ;
#64546=LINE ( 'NONE', #32198, #60822 ) ;
#64552=EDGE_LOOP ( 'NONE', ( #38726, #13484, #3090, #447 ) ) ;
#64555=EDGE_CURVE ( 'NONE', #19369, #30210, #22769, .T. ) ;
#64575=FACE_BOUND ( 'NONE', #30503, .T. ) ;
#64578=AXIS2_PLACEMENT_3D ( 'NONE', #9324, #13909, #55154 ) ;
#64597=CARTESIAN_POINT ( 'NONE',  ( -7.329206686002009974E-14, -46.66904755831211560, 85.00100000000000477 ) ) ;
#64616=EDGE_CURVE ( 'NONE', #19565, #23144, #61451, .T. ) ;
#64623=LINE ( 'NONE', #48083, #27462 ) ;
#64630=VECTOR ( 'NONE', #3442, 1000.000000000000000 ) ;
#64641=VECTOR ( 'NONE', #22572, 1000.000000000000000 ) ;
#64652=LINE ( 'NONE', #54415, #60348 ) ;
#64665=CARTESIAN_POINT ( 'NONE',  ( 0.000000000000000000, 0.000000000000000000, 17.57656211871651308 ) ) ;
#64679=FACE_OUTER_BOUND ( 'NONE', #45820, .T. ) ;
#64711=EDGE_CURVE ( 'NONE', #26921, #24137, #67776, .T. ) ;
#64712=ORIENTED_EDGE ( 'NONE', *, *, #16655, .T. ) ;
#64713=ADVANCED_FACE ( 'NONE', ( #36106 ), #46996, .F. ) ;
#64732=DIRECTION ( 'NONE',  ( 1.000000000000000000, 0.000000000000000000, 0.000000000000000000 ) ) ;
#64748=LINE ( 'NONE', #12675, #22713 ) ;
#64755=DIRECTION ( 'NONE',  ( -0.000000000000000000, -1.000000000000000000, -0.000000000000000000 ) ) ;
#64778=CARTESIAN_POINT ( 'NONE',  ( -46.66904755831210139, 6.635317295611287136E-14, 2.000000000000001776 ) ) ;
#64790=EDGE_CURVE ( 'NONE', #64201, #22983, #7985, .T. ) ;
#64794=LINE ( 'NONE', #44017, #56320 ) ;
#64795=VECTOR ( 'NONE', #1729, 1000.000000000000000 ) ;
#64800=ORIENTED_EDGE ( 'NONE', *, *, #27204, .F. ) ;
#64805=DIRECTION ( 'NONE',  ( 1.000000000000000000, 0.000000000000000000, 0.000000000000000000 ) ) ;
#64824=CIRCLE ( 'NONE', #43462, 74.99999999999998579 ) ;
#64835=LINE ( 'NONE', #31529, #8128 ) ;
#64837=VECTOR ( 'NONE', #19366, 1000.000000000000000 ) ;
#64881=AXIS2_PLACEMENT_3D ( 'NONE', #51412, #41192, #67938 ) ;
#64882=CARTESIAN_POINT ( 'NONE',  ( 26.11269837220809364, 20.55634918610396866, 2.000000000000001776 ) ) ;
#64883=LINE ( 'NONE', #38137, #56576 ) ;
#64911=VERTEX_POINT ( 'NONE', #27604 ) ;
#64928=FACE_BOUND ( 'NONE', #21506, .T. ) ;
#64930=AXIS2_PLACEMENT_3D ( 'NONE', #49557, #2106, #28471 ) ;
#64952=DIRECTION ( 'NONE',  ( -0.000000000000000000, -0.000000000000000000, -1.000000000000000000 ) ) ;
#64960=VERTEX_POINT ( 'NONE', #38876 ) ;
#64972=CARTESIAN_POINT ( 'NONE',  ( 15.55634918610400241, -15.55634918610406103, 85.00100000000000477 ) ) ;
#64981=VECTOR ( 'NONE', #44209, 1000.000000000000000 ) ;
#64988=EDGE_CURVE ( 'NONE', #49065, #39103, #22399, .T. ) ;
#65006=DIRECTION ( 'NONE',  ( 0.000000000000000000, -1.000000000000000000, 0.000000000000000000 ) ) ;
#65010=CARTESIAN_POINT ( 'NONE',  ( -15.55634918610400597, 15.55634918610405748, 0.000000000000000000 ) ) ;
#65016=ORIENTED_EDGE ( 'NONE', *, *, #54127, .T. ) ;
#65041=DIRECTION ( 'NONE',  ( -0.000000000000000000, -0.000000000000000000, -1.000000000000000000 ) ) ;
#65065=ORIENTED_EDGE ( 'NONE', *, *, #61497, .T. ) ;
#65076=ORIENTED_EDGE ( 'NONE', *, *, #50807, .F. ) ;
#65111=VECTOR ( 'NONE', #23262, 1000.000000000000000 ) ;
#65178=DIRECTION ( 'NONE',  ( -0.000000000000000000, -0.000000000000000000, -1.000000000000000000 ) ) ;
#65236=VERTEX_POINT ( 'NONE', #37379 ) ;
#65240=DIRECTION ( 'NONE',  ( 1.000000000000000000, 0.000000000000000000, 0.000000000000000000 ) ) ;
#65252=EDGE_CURVE ( 'NONE', #69309, #60552, #37734, .T. ) ;
#65255=FACE_OUTER_BOUND ( 'NONE', #6114, .T. ) ;
#65256=ORIENTED_EDGE ( 'NONE', *, *, #6766, .T. ) ;
#65268=FACE_BOUND ( 'NONE', #54722, .T. ) ;
#65276=EDGE_LOOP ( 'NONE', ( #44669, #67923, #53363, #13508 ) ) ;
#65282=PLANE ( 'NONE',  #46608 ) ;
#65289=VECTOR ( 'NONE', #3307, 1000.000000000000000 ) ;
#65305=CARTESIAN_POINT ( 'NONE',  ( -4.999999999999936939, 31.11269837220806167, 0.000000000000000000 ) ) ;
#65320=ORIENTED_EDGE ( 'NONE', *, *, #40336, .T. ) ;
#65324=DIRECTION ( 'NONE',  ( 0.000000000000000000, 1.000000000000000000, 0.000000000000000000 ) ) ;
#65335=EDGE_LOOP ( 'NONE', ( #10166, #13862, #877, #5667 ) ) ;
#65342=CARTESIAN_POINT ( 'NONE',  ( -4.999999999999936939, 36.11269837220805812, 2.000000000000001776 ) ) ;
#65353=DIRECTION ( 'NONE',  ( 0.000000000000000000, -0.000000000000000000, -1.000000000000000000 ) ) ;
#65360=CARTESIAN_POINT ( 'NONE',  ( 26.11269837220803325, -10.55634918610409656, 85.00100000000000477 ) ) ;
#65364=VERTEX_POINT ( 'NONE', #2539 ) ;
#65365=CARTESIAN_POINT ( 'NONE',  ( -20.55634918610400419, 20.55634918610405748, 2.000000000000001776 ) ) ;
#65366=VECTOR ( 'NONE', #37571, 1000.000000000000000 ) ;
#65379=DIRECTION ( 'NONE',  ( 0.000000000000000000, 0.000000000000000000, 1.000000000000000000 ) ) ;
#65381=CARTESIAN_POINT ( 'NONE',  ( -46.66904755831210139, 6.635317295611287136E-14, 2.000000000000001776 ) ) ;
#65395=LINE ( 'NONE', #32344, #36573 ) ;
#65447=DIRECTION ( 'NONE',  ( -1.000000000000000000, 0.000000000000000000, 0.000000000000000000 ) ) ;
#65451=VECTOR ( 'NONE', #44561, 1000.000000000000000 ) ;
#65452=CARTESIAN_POINT ( 'NONE',  ( -15.55634918610411077, -41.66904755831209428, 2.000000000000001776 ) ) ;
#65461=LINE ( 'NONE', #38725, #27624 ) ;
#65497=CARTESIAN_POINT ( 'NONE',  ( 46.66904755831207297, -10.55634918610412853, 2.000000000000001776 ) ) ;
#65511=AXIS2_PLACEMENT_3D ( 'NONE', #1894, #36956, #37283 ) ;
#65512=EDGE_LOOP ( 'NONE', ( #61418, #28822, #8056, #33189 ) ) ;
#65513=CARTESIAN_POINT ( 'NONE',  ( 6.375108774214766072E-14, 31.11269837220806167, 0.000000000000000000 ) ) ;
#65524=VERTEX_POINT ( 'NONE', #28934 ) ;
#65531=EDGE_CURVE ( 'NONE', #3625, #39103, #63009, .T. ) ;
#65602=CARTESIAN_POINT ( 'NONE',  ( -31.11269837220812207, -31.11269837220801193, 2.000000000000001776 ) ) ;
#65616=CARTESIAN_POINT ( 'NONE',  ( -15.55634918610396866, 36.11269837220808654, 85.00100000000000477 ) ) ;
#65629=FACE_BOUND ( 'NONE', #7751, .T. ) ;
#65647=ORIENTED_EDGE ( 'NONE', *, *, #14825, .T. ) ;
#65658=VECTOR ( 'NONE', #9169, 1000.000000000000000 ) ;
#65715=VERTEX_POINT ( 'NONE', #4954 ) ;
#65717=AXIS2_PLACEMENT_3D ( 'NONE', #15444, #36895, #5222 ) ;
#65730=VERTEX_POINT ( 'NONE', #69318 ) ;
#65751=VECTOR ( 'NONE', #35246, 1000.000000000000000 ) ;
#65784=ORIENTED_EDGE ( 'NONE', *, *, #39582, .F. ) ;
#65800=ORIENTED_EDGE ( 'NONE', *, *, #18197, .F. ) ;
#65817=PLANE ( 'NONE',  #69349 ) ;
#65819=ORIENTED_EDGE ( 'NONE', *, *, #69087, .F. ) ;
#65822=EDGE_LOOP ( 'NONE', ( #993, #32436 ) ) ;
#65835=ORIENTED_EDGE ( 'NONE', *, *, #26708, .F. ) ;
#65842=LINE ( 'NONE', #44358, #62692 ) ;
#65858=EDGE_CURVE ( 'NONE', #5346, #43873, #3073, .T. ) ;
#65861=ORIENTED_EDGE ( 'NONE', *, *, #19401, .F. ) ;
#65865=VECTOR ( 'NONE', #68550, 1000.000000000000000 ) ;
#65869=DIRECTION ( 'NONE',  ( -0.000000000000000000, -0.000000000000000000, -1.000000000000000000 ) ) ;
#65891=DIRECTION ( 'NONE',  ( 1.000000000000000000, -0.000000000000000000, -0.000000000000000000 ) ) ;
#65909=DIRECTION ( 'NONE',  ( 0.000000000000000000, -1.000000000000000000, 0.000000000000000000 ) ) ;
#65940=ORIENTED_EDGE ( 'NONE', *, *, #27929, .F. ) ;
#65977=DIRECTION ( 'NONE',  ( -1.000000000000000000, 0.000000000000000000, 0.000000000000000000 ) ) ;
#65986=DIRECTION ( 'NONE',  ( 1.000000000000000000, 0.000000000000000000, 0.000000000000000000 ) ) ;
#66002=VECTOR ( 'NONE', #12025, 1000.000000000000000 ) ;
#66003=DIRECTION ( 'NONE',  ( -0.000000000000000000, -0.000000000000000000, -1.000000000000000000 ) ) ;
#66016=VECTOR ( 'NONE', #48200, 1000.000000000000000 ) ;
#66033=CARTESIAN_POINT ( 'NONE',  ( 10.55634918610403084, -3.079134169858832593E-14, 2.000000000000001776 ) ) ;
#66046=CARTESIAN_POINT ( 'NONE',  ( -31.11269837220804035, 15.55634918610408945, 0.000000000000000000 ) ) ;
#66064=DIRECTION ( 'NONE',  ( 0.000000000000000000, 0.000000000000000000, 1.000000000000000000 ) ) ;
#66080=FACE_BOUND ( 'NONE', #26398, .T. ) ;
#66148=CARTESIAN_POINT ( 'NONE',  ( 0.000000000000000000, 0.000000000000000000, 85.00000000000000000 ) ) ;
#66157=EDGE_CURVE ( 'NONE', #22868, #56240, #55392, .T. ) ;
#66165=DIRECTION ( 'NONE',  ( 1.000000000000000000, -0.000000000000000000, -0.000000000000000000 ) ) ;
#66166=VERTEX_POINT ( 'NONE', #44850 ) ;
#66189=PLANE ( 'NONE',  #9216 ) ;
#66196=CARTESIAN_POINT ( 'NONE',  ( 41.66904755831208007, -15.55634918610412853, 2.000000000000000000 ) ) ;
#66205=LINE ( 'NONE', #17994, #41150 ) ;
#66210=DIRECTION ( 'NONE',  ( 1.000000000000000000, 0.000000000000000000, 0.000000000000000000 ) ) ;
#66232=VECTOR ( 'NONE', #4547, 1000.000000000000000 ) ;
#66241=LINE ( 'NONE', #49669, #31910 ) ;
#66242=CARTESIAN_POINT ( 'NONE',  ( 7.762887554996211747E-14, 46.66904755831208718, 2.000000000000001776 ) ) ;
#66244=EDGE_LOOP ( 'NONE', ( #20109, #40435, #51685, #54956 ) ) ;
#66278=FACE_OUTER_BOUND ( 'NONE', #11258, .T. ) ;
#66287=LINE ( 'NONE', #27221, #31504 ) ;
#66308=CARTESIAN_POINT ( 'NONE',  ( -15.55634918610403439, 2.818925648462311528E-14, 85.00100000000000477 ) ) ;
#66317=PLANE ( 'NONE',  #12115 ) ;
#66342=LINE ( 'NONE', #13548, #39282 ) ;
#66345=EDGE_CURVE ( 'NONE', #50424, #62726, #2213, .T. ) ;
#66351=ORIENTED_EDGE ( 'NONE', *, *, #40417, .F. ) ;
#66370=DIRECTION ( 'NONE',  ( -1.000000000000000000, 0.000000000000000000, 0.000000000000000000 ) ) ;
#66419=ORIENTED_EDGE ( 'NONE', *, *, #13497, .F. ) ;
#66423=LINE ( 'NONE', #65010, #28190 ) ;
#66434=VECTOR ( 'NONE', #39845, 1000.000000000000000 ) ;
#66455=CARTESIAN_POINT ( 'NONE',  ( 26.11269837220803325, -15.55634918610409656, 85.00100000000000477 ) ) ;
#66473=VECTOR ( 'NONE', #6751, 1000.000000000000000 ) ;
#66496=VERTEX_POINT ( 'NONE', #18729 ) ;
#66516=ORIENTED_EDGE ( 'NONE', *, *, #16349, .T. ) ;
#66542=CARTESIAN_POINT ( 'NONE',  ( 10.55634918610409656, 31.11269837220803325, 2.000000000000001776 ) ) ;
#66552=CARTESIAN_POINT ( 'NONE',  ( -46.66904755831210139, 6.635317295611287136E-14, 2.000000000000001776 ) ) ;
#66553=ADVANCED_FACE ( 'NONE', ( #24364 ), #61973, .F. ) ;
#66566=ORIENTED_EDGE ( 'NONE', *, *, #50161, .F. ) ;
#66578=CARTESIAN_POINT ( 'NONE',  ( -36.11269837220804391, 15.55634918610408945, 2.000000000000001776 ) ) ;
#66580=VECTOR ( 'NONE', #44963, 1000.000000000000000 ) ;
#66598=LINE ( 'NONE', #18386, #66434 ) ;
#66608=PLANE ( 'NONE',  #52775 ) ;
#66645=ADVANCED_FACE ( 'NONE', ( #57748 ), #33085, .F. ) ;
#66650=EDGE_CURVE ( 'NONE', #17510, #1454, #21821, .T. ) ;
#66664=CARTESIAN_POINT ( 'NONE',  ( 10.55634918610411432, 46.66904755831205875, 2.000000000000001776 ) ) ;
#66667=ORIENTED_EDGE ( 'NONE', *, *, #5444, .T. ) ;
#66687=ORIENTED_EDGE ( 'NONE', *, *, #58801, .T. ) ;
#66696=CARTESIAN_POINT ( 'NONE',  ( 41.66904755831208007, -15.55634918610412853, 85.00100000000000477 ) ) ;
#66708=CARTESIAN_POINT ( 'NONE',  ( 2.905661822261151883E-14, 15.55634918610403084, 85.00100000000000477 ) ) ;
#66714=VECTOR ( 'NONE', #65869, 1000.000000000000000 ) ;
#66744=LINE ( 'NONE', #1656, #6176 ) ;
#66772=LINE ( 'NONE', #20534, #9366 ) ;
#66773=FACE_BOUND ( 'NONE', #55379, .T. ) ;
#66778=CONICAL_SURFACE ( 'NONE', #25204, 73.43826238111391547, 0.6747409422235518539 ) ;
#66781=VECTOR ( 'NONE', #47421, 1000.000000000000000 ) ;
#66796=ORIENTED_EDGE ( 'NONE', *, *, #15404, .T. ) ;
#66813=LINE ( 'NONE', #57627, #14884 ) ;
#66816=VERTEX_POINT ( 'NONE', #23582 ) ;
#66817=DIRECTION ( 'NONE',  ( -0.000000000000000000, -0.000000000000000000, -1.000000000000000000 ) ) ;
#66832=AXIS2_PLACEMENT_3D ( 'NONE', #50530, #44558, #8319 ) ;
#66835=VECTOR ( 'NONE', #67108, 1000.000000000000000 ) ;
#66897=EDGE_LOOP ( 'NONE', ( #12729, #25960, #68959, #68694 ) ) ;
#66899=DIRECTION ( 'NONE',  ( 0.000000000000000000, 0.000000000000000000, -1.000000000000000000 ) ) ;
#66929=DIRECTION ( 'NONE',  ( -0.000000000000000000, -0.000000000000000000, -1.000000000000000000 ) ) ;
#66940=ORIENTED_EDGE ( 'NONE', *, *, #33510, .F. ) ;
#66955=CARTESIAN_POINT ( 'NONE',  ( -15.55634918610411077, -46.66904755831208718, 85.00100000000000477 ) ) ;
#66958=ADVANCED_FACE ( 'NONE', ( #20036 ), #25668, .F. ) ;
#66968=PLANE ( 'NONE',  #11365 ) ;
#66970=EDGE_CURVE ( 'NONE', #33219, #11967, #60270, .T. ) ;
#66981=AXIS2_PLACEMENT_3D ( 'NONE', #33462, #39084, #60524 ) ;
#66998=PLANE ( 'NONE',  #40797 ) ;
#67006=CARTESIAN_POINT ( 'NONE',  ( -31.11269837220809364, -15.55634918610397754, 85.00100000000000477 ) ) ;
#67016=LINE ( 'NONE', #51170, #10001 ) ;
#67027=EDGE_CURVE ( 'NONE', #10200, #32423, #36210, .T. ) ;
#67031=EDGE_CURVE ( 'NONE', #59604, #54421, #69242, .T. ) ;
#67042=CARTESIAN_POINT ( 'NONE',  ( 10.55634918610409656, 36.11269837220803680, 0.000000000000000000 ) ) ;
#67050=ORIENTED_EDGE ( 'NONE', *, *, #63366, .T. ) ;
#67059=DIRECTION ( 'NONE',  ( -0.000000000000000000, -0.000000000000000000, -1.000000000000000000 ) ) ;
#67069=DIRECTION ( 'NONE',  ( 0.000000000000000000, 1.000000000000000000, -0.000000000000000000 ) ) ;
#67070=AXIS2_PLACEMENT_3D ( 'NONE', #5194, #20329, #69542 ) ;
#67080=ORIENTED_EDGE ( 'NONE', *, *, #26096, .F. ) ;
#67100=ORIENTED_EDGE ( 'NONE', *, *, #3981, .F. ) ;
#67102=ORIENTED_EDGE ( 'NONE', *, *, #66650, .F. ) ;
#67108=DIRECTION ( 'NONE',  ( 0.000000000000000000, 1.000000000000000000, -0.000000000000000000 ) ) ;
#67114=EDGE_LOOP ( 'NONE', ( #66516, #9686, #69133, #66351 ) ) ;
#67124=FACE_BOUND ( 'NONE', #67586, .T. ) ;
#67125=CIRCLE ( 'NONE', #53566, 65.00000000000000000 ) ;
#67129=EDGE_CURVE ( 'NONE', #192, #22403, #2504, .T. ) ;
#67139=CARTESIAN_POINT ( 'NONE',  ( -2.645453300864630819E-14, -10.55634918610403439, 85.00100000000000477 ) ) ;
#67151=EDGE_LOOP ( 'NONE', ( #46265, #41729, #30007, #9948 ) ) ;
#67164=LINE ( 'NONE', #36167, #64294 ) ;
#67168=ORIENTED_EDGE ( 'NONE', *, *, #68839, .T. ) ;
#67186=ORIENTED_EDGE ( 'NONE', *, *, #54960, .F. ) ;
#67234=VECTOR ( 'NONE', #24129, 1000.000000000000000 ) ;
#67242=CARTESIAN_POINT ( 'NONE',  ( 15.55634918610396511, -46.66904755831214402, 85.00100000000000477 ) ) ;
#67245=CARTESIAN_POINT ( 'NONE',  ( -73.43826238111391547, 8.993593295997464589E-15, 26.24939009510892518 ) ) ;
#67248=DIRECTION ( 'NONE',  ( -0.000000000000000000, -0.000000000000000000, -1.000000000000000000 ) ) ;
#67265=LINE ( 'NONE', #56687, #9803 ) ;
#67273=EDGE_LOOP ( 'NONE', ( #55484, #37949, #25585, #59995 ) ) ;
#67275=LINE ( 'NONE', #66578, #63090 ) ;
#67286=ORIENTED_EDGE ( 'NONE', *, *, #63136, .T. ) ;
#67309=ORIENTED_EDGE ( 'NONE', *, *, #14830, .F. ) ;
#67347=LINE ( 'NONE', #25474, #1888 ) ;
#67362=EDGE_CURVE ( 'NONE', #25726, #35180, #66772, .T. ) ;
#67368=CARTESIAN_POINT ( 'NONE',  ( -20.55634918610405748, -15.55634918610400774, 85.00100000000000477 ) ) ;
#67373=PLANE ( 'NONE',  #24248 ) ;
#67388=VERTEX_POINT ( 'NONE', #16642 ) ;
#67394=CARTESIAN_POINT ( 'NONE',  ( 15.55634918610406103, 15.55634918610400241, 2.000000000000001776 ) ) ;
#67403=DIRECTION ( 'NONE',  ( -0.000000000000000000, -0.000000000000000000, -1.000000000000000000 ) ) ;
#67432=EDGE_CURVE ( 'NONE', #64960, #11163, #34233, .T. ) ;
#67438=VECTOR ( 'NONE', #57784, 1000.000000000000000 ) ;
#67439=EDGE_CURVE ( 'NONE', #38815, #13387, #11712, .T. ) ;
#67446=ORIENTED_EDGE ( 'NONE', *, *, #45966, .F. ) ;
#67457=FACE_BOUND ( 'NONE', #39864, .T. ) ;
#67475=CARTESIAN_POINT ( 'NONE',  ( -5.000000000000026645, -15.55634918610403616, 0.000000000000000000 ) ) ;
#67479=VERTEX_POINT ( 'NONE', #39164 ) ;
#67482=DIRECTION ( 'NONE',  ( -1.000000000000000000, 0.000000000000000000, 0.000000000000000000 ) ) ;
#67491=CARTESIAN_POINT ( 'NONE',  ( -4.999999999999971578, 15.55634918610403084, 2.000000000000001776 ) ) ;
#67581=DIRECTION ( 'NONE',  ( 0.000000000000000000, 0.000000000000000000, 1.000000000000000000 ) ) ;
#67586=EDGE_LOOP ( 'NONE', ( #4316, #64009, #50324, #59524 ) ) ;
#67602=ORIENTED_EDGE ( 'NONE', *, *, #56361, .F. ) ;
#67619=ADVANCED_FACE ( 'NONE', ( #29923 ), #60884, .F. ) ;
#67643=EDGE_LOOP ( 'NONE', ( #61467, #43741, #44965, #21263 ) ) ;
#67645=ORIENTED_EDGE ( 'NONE', *, *, #27694, .T. ) ;
#67660=ORIENTED_EDGE ( 'NONE', *, *, #1349, .T. ) ;
#67670=FACE_OUTER_BOUND ( 'NONE', #21835, .T. ) ;
#67694=CARTESIAN_POINT ( 'NONE',  ( -46.66904755831212981, -10.55634918610397222, 2.000000000000001776 ) ) ;
#67696=ORIENTED_EDGE ( 'NONE', *, *, #65858, .F. ) ;
#67701=CARTESIAN_POINT ( 'NONE',  ( -66.50000000000000000, 8.143901214329899974E-15, -0.002000000000002000178 ) ) ;
#67723=LINE ( 'NONE', #56459, #31660 ) ;
#67757=CARTESIAN_POINT ( 'NONE',  ( 26.11269837220812562, 31.11269837220800483, 2.000000000000000000 ) ) ;
#67770=PLANE ( 'NONE',  #14383 ) ;
#67773=AXIS2_PLACEMENT_3D ( 'NONE', #15718, #54013, #58275 ) ;
#67776=LINE ( 'NONE', #35764, #11143 ) ;
#67783=LINE ( 'NONE', #8348, #54110 ) ;
#67789=VERTEX_POINT ( 'NONE', #25352 ) ;
#67791=ORIENTED_EDGE ( 'NONE', *, *, #35206, .F. ) ;
#67824=EDGE_LOOP ( 'NONE', ( #45771, #27345, #17450, #14042 ) ) ;
#67838=VERTEX_POINT ( 'NONE', #9159 ) ;
#67841=CARTESIAN_POINT ( 'NONE',  ( -46.66904755831210139, 5.000000000000066613, 0.000000000000000000 ) ) ;
#67851=ORIENTED_EDGE ( 'NONE', *, *, #632, .T. ) ;
#67858=ORIENTED_EDGE ( 'NONE', *, *, #29092, .T. ) ;
#67865=VERTEX_POINT ( 'NONE', #59052 ) ;
#67867=DIRECTION ( 'NONE',  ( -0.000000000000000000, -0.000000000000000000, -1.000000000000000000 ) ) ;
#67900=PLANE ( 'NONE',  #58695 ) ;
#67901=DIRECTION ( 'NONE',  ( -0.000000000000000000, -0.000000000000000000, -1.000000000000000000 ) ) ;
#67906=EDGE_CURVE ( 'NONE', #56869, #65730, #43566, .T. ) ;
#67923=ORIENTED_EDGE ( 'NONE', *, *, #35646, .F. ) ;
#67926=EDGE_LOOP ( 'NONE', ( #25052, #64335, #68600, #5852 ) ) ;
#67934=CARTESIAN_POINT ( 'NONE',  ( -20.55634918610400419, 15.55634918610405748, 85.00100000000000477 ) ) ;
#67938=DIRECTION ( 'NONE',  ( 1.000000000000000000, 0.000000000000000000, 0.000000000000000000 ) ) ;
#67959=VECTOR ( 'NONE', #56903, 1000.000000000000000 ) ;
#67973=EDGE_CURVE ( 'NONE', #24549, #36560, #54817, .T. ) ;
#67980=ORIENTED_EDGE ( 'NONE', *, *, #55443, .T. ) ;
#68009=ORIENTED_EDGE ( 'NONE', *, *, #59389, .F. ) ;
#68013=CARTESIAN_POINT ( 'NONE',  ( -5.000000000000000000, 5.000000000000000000, 0.000000000000000000 ) ) ;
#68024=DIRECTION ( 'NONE',  ( -0.000000000000000000, -0.000000000000000000, -1.000000000000000000 ) ) ;
#68033=PLANE ( 'NONE',  #28278 ) ;
#68039=ORIENTED_EDGE ( 'NONE', *, *, #54850, .F. ) ;
#68045=CARTESIAN_POINT ( 'NONE',  ( 15.55634918610409656, 31.11269837220803325, 2.000000000000001776 ) ) ;
#68090=DIRECTION ( 'NONE',  ( 1.000000000000000000, -0.000000000000000000, 0.000000000000000000 ) ) ;
#68128=CARTESIAN_POINT ( 'NONE',  ( 2.905661822261151883E-14, 20.55634918610402906, 85.00100000000000477 ) ) ;
#68139=ORIENTED_EDGE ( 'NONE', *, *, #3344, .T. ) ;
#68151=FACE_BOUND ( 'NONE', #8368, .T. ) ;
#68164=CARTESIAN_POINT ( 'NONE',  ( 15.55634918610409656, 31.11269837220803325, 2.000000000000001776 ) ) ;
#68189=EDGE_LOOP ( 'NONE', ( #48951, #64114, #53029, #45051 ) ) ;
#68196=ORIENTED_EDGE ( 'NONE', *, *, #49399, .T. ) ;
#68200=DIRECTION ( 'NONE',  ( 1.000000000000000000, 0.000000000000000000, 0.000000000000000000 ) ) ;
#68225=EDGE_LOOP ( 'NONE', ( #63008, #4472, #42510, #32355 ) ) ;
#68230=ORIENTED_EDGE ( 'NONE', *, *, #47316, .T. ) ;
#68256=VECTOR ( 'NONE', #29248, 1000.000000000000000 ) ;
#68266=ORIENTED_EDGE ( 'NONE', *, *, #31755, .F. ) ;
#68284=CARTESIAN_POINT ( 'NONE',  ( -20.55634918610408945, -26.11269837220804035, 85.00100000000000477 ) ) ;
#68372=CARTESIAN_POINT ( 'NONE',  ( -15.55634918610408945, -26.11269837220804035, 85.00100000000000477 ) ) ;
#68376=LINE ( 'NONE', #35678, #13132 ) ;
#68387=EDGE_CURVE ( 'NONE', #11547, #34612, #9946, .T. ) ;
#68402=VERTEX_POINT ( 'NONE', #20485 ) ;
#68405=EDGE_CURVE ( 'NONE', #48270, #30095, #15217, .T. ) ;
#68406=VECTOR ( 'NONE', #42901, 1000.000000000000000 ) ;
#68411=EDGE_CURVE ( 'NONE', #17896, #42033, #4326, .T. ) ;
#68416=CARTESIAN_POINT ( 'NONE',  ( -46.66904755831210139, 6.635317295611287136E-14, 0.000000000000000000 ) ) ;
#68418=ORIENTED_EDGE ( 'NONE', *, *, #28463, .T. ) ;
#68481=VECTOR ( 'NONE', #42616, 1000.000000000000000 ) ;
#68482=CARTESIAN_POINT ( 'NONE',  ( 0.000000000000000000, 0.000000000000000000, 0.000000000000000000 ) ) ;
#68483=ORIENTED_EDGE ( 'NONE', *, *, #7661, .F. ) ;
#68489=CARTESIAN_POINT ( 'NONE',  ( 31.11269837220806522, 4.999999999999936939, 2.000000000000001776 ) ) ;
#68490=EDGE_LOOP ( 'NONE', ( #23526, #35858, #3198, #36059 ) ) ;
#68550=DIRECTION ( 'NONE',  ( 1.000000000000000000, -0.000000000000000000, -0.000000000000000000 ) ) ;
#68563=DIRECTION ( 'NONE',  ( -1.000000000000000000, 0.000000000000000000, 0.000000000000000000 ) ) ;
#68583=CARTESIAN_POINT ( 'NONE',  ( -65.00000000000000000, 7.960204194457797252E-15, 85.00000000000000000 ) ) ;
#68589=ORIENTED_EDGE ( 'NONE', *, *, #13575, .F. ) ;
#68600=ORIENTED_EDGE ( 'NONE', *, *, #25887, .T. ) ;
#68632=LINE ( 'NONE', #13787, #65751 ) ;
#68656=CARTESIAN_POINT ( 'NONE',  ( 26.11269837220812562, 31.11269837220800483, 85.00100000000000477 ) ) ;
#68671=DIRECTION ( 'NONE',  ( 0.000000000000000000, -1.000000000000000000, 0.000000000000000000 ) ) ;
#68683=EDGE_CURVE ( 'NONE', #26889, #38519, #42964, .T. ) ;
#68694=ORIENTED_EDGE ( 'NONE', *, *, #18763, .T. ) ;
#68697=VECTOR ( 'NONE', #349, 1000.000000000000000 ) ;
#68698=LINE ( 'NONE', #68372, #15040 ) ;
#68721=LINE ( 'NONE', #36382, #40190 ) ;
#68733=DIRECTION ( 'NONE',  ( -0.000000000000000000, -0.000000000000000000, -1.000000000000000000 ) ) ;
#68734=DIRECTION ( 'NONE',  ( -0.000000000000000000, -0.000000000000000000, -1.000000000000000000 ) ) ;
#68750=ORIENTED_EDGE ( 'NONE', *, *, #1909, .F. ) ;
#68752=ORIENTED_EDGE ( 'NONE', *, *, #36534, .T. ) ;
#68792=LINE ( 'NONE', #36113, #45462 ) ;
#68815=CYLINDRICAL_SURFACE ( 'NONE', #34836, 74.99999999999998579 ) ;
#68830=ORIENTED_EDGE ( 'NONE', *, *, #43108, .T. ) ;
#68839=EDGE_CURVE ( 'NONE', #37709, #38638, #41525, .T. ) ;
#68858=AXIS2_PLACEMENT_3D ( 'NONE', #18160, #55081, #33994 ) ;
#68861=CARTESIAN_POINT ( 'NONE',  ( 15.55634918610406103, 15.55634918610400241, 85.00100000000000477 ) ) ;
#68881=PLANE ( 'NONE',  #65717 ) ;
#68882=VECTOR ( 'NONE', #14203, 1000.000000000000000 ) ;
#68887=DIRECTION ( 'NONE',  ( 0.000000000000000000, 0.000000000000000000, 1.000000000000000000 ) ) ;
#68900=AXIS2_PLACEMENT_3D ( 'NONE', #91, #43687, #21892 ) ;
#68902=CARTESIAN_POINT ( 'NONE',  ( -31.11269837220806878, 5.594483210025202879E-14, 2.000000000000001776 ) ) ;
#68944=VECTOR ( 'NONE', #61606, 1000.000000000000000 ) ;
#68947=VECTOR ( 'NONE', #63413, 1000.000000000000000 ) ;
#68959=ORIENTED_EDGE ( 'NONE', *, *, #28369, .T. ) ;
#68972=ADVANCED_FACE ( 'NONE', ( #16160 ), #11223, .F. ) ;
#68977=LINE ( 'NONE', #42602, #46019 ) ;
#69014=VERTEX_POINT ( 'NONE', #54474 ) ;
#69032=CARTESIAN_POINT ( 'NONE',  ( 15.55634918610400241, -15.55634918610406103, 2.000000000000001776 ) ) ;
#69033=LINE ( 'NONE', #48603, #33214 ) ;
#69043=ORIENTED_EDGE ( 'NONE', *, *, #3173, .F. ) ;
#69066=EDGE_CURVE ( 'NONE', #39519, #11058, #37516, .T. ) ;
#69076=LINE ( 'NONE', #68416, #60992 ) ;
#69086=EDGE_CURVE ( 'NONE', #48274, #31799, #6301, .T. ) ;
#69087=EDGE_CURVE ( 'NONE', #18908, #4486, #5600, .T. ) ;
#69096=VECTOR ( 'NONE', #30936, 1000.000000000000000 ) ;
#69111=LINE ( 'NONE', #53955, #7055 ) ;
#69133=ORIENTED_EDGE ( 'NONE', *, *, #48469, .F. ) ;
#69149=ORIENTED_EDGE ( 'NONE', *, *, #5851, .T. ) ;
#69169=ORIENTED_EDGE ( 'NONE', *, *, #12497, .T. ) ;
#69185=VECTOR ( 'NONE', #62623, 1000.000000000000000 ) ;
#69237=EDGE_CURVE ( 'NONE', #17852, #29447, #56228, .T. ) ;
#69238=VECTOR ( 'NONE', #41186, 1000.000000000000000 ) ;
#69242=LINE ( 'NONE', #3856, #40652 ) ;
#69246=ORIENTED_EDGE ( 'NONE', *, *, #51299, .T. ) ;
#69247=ORIENTED_EDGE ( 'NONE', *, *, #52411, .T. ) ;
#69270=CARTESIAN_POINT ( 'NONE',  ( -31.11269837220801193, 31.11269837220812207, 85.00100000000000477 ) ) ;
#69271=ORIENTED_EDGE ( 'NONE', *, *, #22627, .T. ) ;
#69308=EDGE_CURVE ( 'NONE', #42408, #1617, #26306, .T. ) ;
#69309=VERTEX_POINT ( 'NONE', #30541 ) ;
#69318=CARTESIAN_POINT ( 'NONE',  ( -4.999999999999971578, 15.55634918610403084, 0.000000000000000000 ) ) ;
#69321=ORIENTED_EDGE ( 'NONE', *, *, #32971, .T. ) ;
#69349=AXIS2_PLACEMENT_3D ( 'NONE', #34846, #23592, #17964 ) ;
#69375=LINE ( 'NONE', #20843, #19551 ) ;
#69387=ADVANCED_FACE ( 'NONE', ( #36508 ), #9781, .F. ) ;
#69388=FACE_OUTER_BOUND ( 'NONE', #67151, .T. ) ;
#69397=FACE_OUTER_BOUND ( 'NONE', #52299, .T. ) ;
#69408=CARTESIAN_POINT ( 'NONE',  ( 31.11269837220806522, 4.999999999999936939, 85.00100000000000477 ) ) ;
#69409=CARTESIAN_POINT ( 'NONE',  ( -15.55634918610411077, -41.66904755831209428, 0.000000000000000000 ) ) ;
#69424=LINE ( 'NONE', #53229, #44456 ) ;
#69427=ORIENTED_EDGE ( 'NONE', *, *, #36076, .F. ) ;
#69428=CARTESIAN_POINT ( 'NONE',  ( -51.66904755831212981, -15.55634918610397222, 2.000000000000000000 ) ) ;
#69435=CARTESIAN_POINT ( 'NONE',  ( 46.66904755831210139, 4.999999999999909406, 2.000000000000001776 ) ) ;
#69444=ADVANCED_FACE ( 'NONE', ( #63929 ), #6573, .F. ) ;
#69494=FACE_BOUND ( 'NONE', #58854, .T. ) ;
#69499=DIRECTION ( 'NONE',  ( 0.000000000000000000, 1.000000000000000000, 0.000000000000000000 ) ) ;
#69508=ORIENTED_EDGE ( 'NONE', *, *, #12189, .F. ) ;
#69509=ORIENTED_EDGE ( 'NONE', *, *, #50654, .T. ) ;
#69531=LINE ( 'NONE', #59928, #54683 ) ;
#69532=CARTESIAN_POINT ( 'NONE',  ( -31.11269837220809364, -10.55634918610397932, 85.00100000000000477 ) ) ;
#69534=VECTOR ( 'NONE', #39994, 1000.000000000000000 ) ;
#69542=DIRECTION ( 'NONE',  ( 0.000000000000000000, 0.000000000000000000, 1.000000000000000000 ) ) ;
#69564=CARTESIAN_POINT ( 'NONE',  ( -20.55634918610405748, -15.55634918610400774, 85.00100000000000477 ) ) ;
#69565=LINE ( 'NONE', #59016, #65865 ) ;
ENDSEC;
END-ISO-10303-21;
